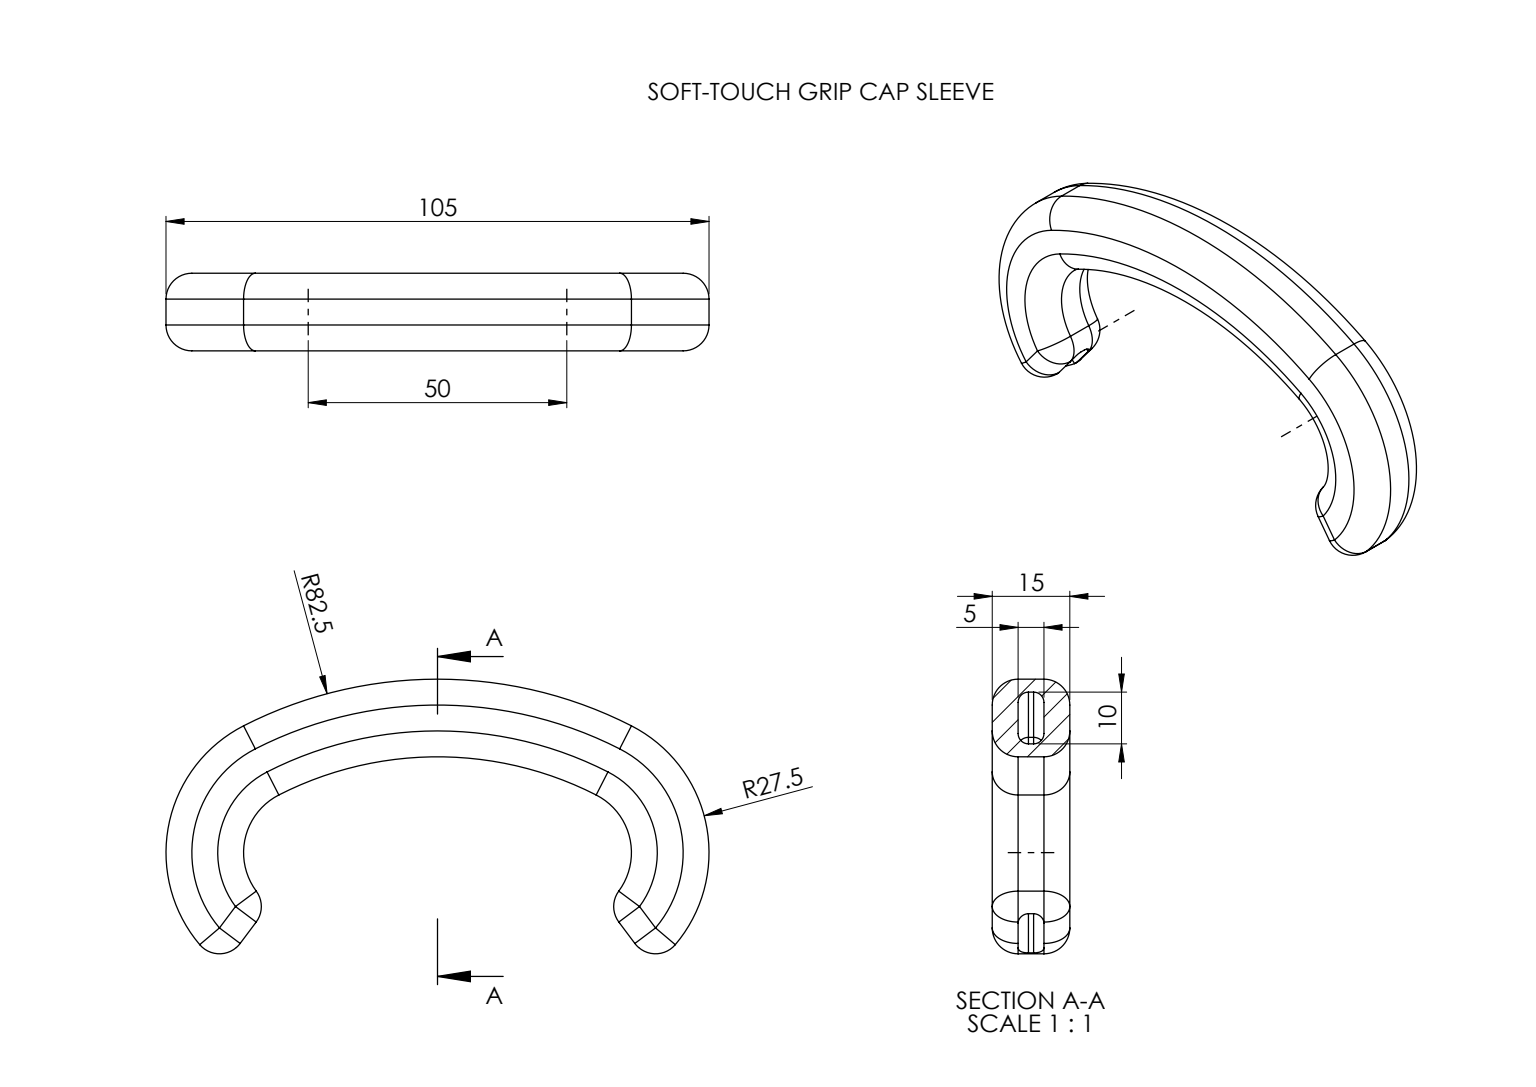
ISO-10303-21;
HEADER;
FILE_DESCRIPTION (('STEP AP214'),
    '1' );
FILE_NAME ('Soft-Touch Grip Cap Sleeve.step',
    '2026-10-08T14:03:35',
    ( '' ),
    ( '' ),
    'SwSTEP 2.0',
    'SolidWorks 2026',
    '' );
FILE_SCHEMA (( 'AUTOMOTIVE_DESIGN' ));
ENDSEC;

DATA;
#11=ORIENTED_EDGE ( 'NONE', *, *, #6966, .F. ) ;
#15=CARTESIAN_POINT ( 'NONE',  ( 35.45454545454547457, 140.4866414850956460, 0.5000000000000000000 ) ) ;
#29=AXIS2_PLACEMENT_3D ( 'NONE', #13329, #9153, #677 ) ;
#40=DIRECTION ( 'NONE',  ( 1.000000000000000000, 8.163404592832038896E-16, 0.000000000000000000 ) ) ;
#44=AXIS2_PLACEMENT_3D ( 'NONE', #13672, #4217, #12871 ) ;
#50=ORIENTED_EDGE ( 'NONE', *, *, #9118, .T. ) ;
#55=B_SPLINE_CURVE_WITH_KNOTS ( 'NONE', 3,
 ( #12024, #7964, #3604, #11191, #2412, #1580, #5937, #3460, #13327, #5788, #331, #6692, #3526, #3678, #4586, #9152 ),
 .UNSPECIFIED., .F., .F.,
 ( 4, 2, 2, 2, 2, 2, 2, 4 ),
 ( 1.967444805616585729E-07, 0.0004077652619395022980, 0.0008153337793984429286, 0.001630470814316324190, 0.002038039331775264550, 0.002445607849234205343, 0.002853176366693145703, 0.003260744884152086496 ),
 .UNSPECIFIED. ) ;
#56=FACE_OUTER_BOUND ( 'NONE', #8177, .T. ) ;
#63=ORIENTED_EDGE ( 'NONE', *, *, #3775, .F. ) ;
#71=ADVANCED_FACE ( 'NONE', ( #7311 ), #13694, .F. ) ;
#72=ORIENTED_EDGE ( 'NONE', *, *, #13139, .F. ) ;
#94=DIRECTION ( 'NONE',  ( 0.000000000000000000, 0.000000000000000000, 1.000000000000000000 ) ) ;
#105=LINE ( 'NONE', #1342, #981 ) ;
#108=CARTESIAN_POINT ( 'NONE',  ( 39.99999999999999289, 120.0000000000000142, -0.5000000000000000000 ) ) ;
#110=ORIENTED_EDGE ( 'NONE', *, *, #13403, .F. ) ;
#115=DIRECTION ( 'NONE',  ( 0.000000000000000000, 0.000000000000000000, 1.000000000000000000 ) ) ;
#121=AXIS2_PLACEMENT_3D ( 'NONE', #813, #875, #8370 ) ;
#138=CARTESIAN_POINT ( 'NONE',  ( -49.99999999999999289, 120.0000000000000142, -0.5000000000000000000 ) ) ;
#139=EDGE_CURVE ( 'NONE', #6890, #1913, #9510, .T. ) ;
#140=FACE_OUTER_BOUND ( 'NONE', #958, .T. ) ;
#148=ORIENTED_EDGE ( 'NONE', *, *, #400, .T. ) ;
#152=DIRECTION ( 'NONE',  ( 1.000000000000000000, 0.000000000000000000, 0.000000000000000000 ) ) ;
#177=ORIENTED_EDGE ( 'NONE', *, *, #6787, .T. ) ;
#187=DIRECTION ( 'NONE',  ( -1.000000000000000000, 0.000000000000000000, 0.000000000000000000 ) ) ;
#196=CARTESIAN_POINT ( 'NONE',  ( 0.000000000000000000, 71.01020514433645303, 7.500000000000000000 ) ) ;
#206=AXIS2_PLACEMENT_3D ( 'NONE', #6163, #5168, #5231 ) ;
#214=VERTEX_POINT ( 'NONE', #5795 ) ;
#224=AXIS2_PLACEMENT_3D ( 'NONE', #10271, #2564, #8106 ) ;
#225=ORIENTED_EDGE ( 'NONE', *, *, #6865, .T. ) ;
#245=AXIS2_PLACEMENT_3D ( 'NONE', #10275, #9294, #13478 ) ;
#272=ORIENTED_EDGE ( 'NONE', *, *, #8857, .F. ) ;
#273=CARTESIAN_POINT ( 'NONE',  ( 35.22727272727274794, 140.0412797136805523, 2.499999999999999556 ) ) ;
#281=EDGE_LOOP ( 'NONE', ( #6165, #11619, #12587 ) ) ;
#289=EDGE_CURVE ( 'NONE', #6878, #1278, #2220, .T. ) ;
#298=AXIS2_PLACEMENT_3D ( 'NONE', #1298, #13105, #6426 ) ;
#303=EDGE_LOOP ( 'NONE', ( #1188, #1446, #12340 ) ) ;
#316=AXIS2_PLACEMENT_3D ( 'NONE', #6986, #3754, #479 ) ;
#330=DIRECTION ( 'NONE',  ( -0.4545454545454531425, -0.8907235428302472391, 0.000000000000000000 ) ) ;
#331=CARTESIAN_POINT ( 'NONE',  ( -39.64259366921353944, 101.1295926276828396, -2.298140577494256931 ) ) ;
#347=AXIS2_PLACEMENT_3D ( 'NONE', #5420, #4428, #2399 ) ;
#351=ORIENTED_EDGE ( 'NONE', *, *, #9753, .F. ) ;
#355=ORIENTED_EDGE ( 'NONE', *, *, #4560, .T. ) ;
#362=AXIS2_PLACEMENT_3D ( 'NONE', #3358, #4277, #12857 ) ;
#365=DIRECTION ( 'NONE',  ( 0.000000000000000000, 0.000000000000000000, 1.000000000000000000 ) ) ;
#369=VERTEX_POINT ( 'NONE', #1786 ) ;
#370=VECTOR ( 'NONE', #9228, 1000.000000000000000 ) ;
#377=DIRECTION ( 'NONE',  ( 0.000000000000000000, 0.000000000000000000, 1.000000000000000000 ) ) ;
#379=EDGE_LOOP ( 'NONE', ( #6863, #5264, #11175, #13440 ) ) ;
#381=AXIS2_PLACEMENT_3D ( 'NONE', #9717, #9650, #7739 ) ;
#382=DIRECTION ( 'NONE',  ( 1.000000000000000000, 0.000000000000000000, 0.000000000000000000 ) ) ;
#397=VERTEX_POINT ( 'NONE', #7385 ) ;
#400=EDGE_CURVE ( 'NONE', #6752, #9552, #11414, .T. ) ;
#406=EDGE_CURVE ( 'NONE', #397, #11234, #4095, .T. ) ;
#410=DIRECTION ( 'NONE',  ( 0.000000000000000000, 0.000000000000000000, 1.000000000000000000 ) ) ;
#414=CARTESIAN_POINT ( 'NONE',  ( 39.06230589874904524, 109.5835921350012683, 2.499999999999999556 ) ) ;
#422=CARTESIAN_POINT ( 'NONE',  ( -39.31777158827905794, 101.3359913474317011, 2.434761661425243418 ) ) ;
#429=DIRECTION ( 'NONE',  ( 0.000000000000000000, 0.000000000000000000, 1.000000000000000000 ) ) ;
#435=VECTOR ( 'NONE', #12367, 1000.000000000000000 ) ;
#436=CARTESIAN_POINT ( 'NONE',  ( -34.25812584745457201, 108.1980041606221192, -0.5000000000000000000 ) ) ;
#448=EDGE_CURVE ( 'NONE', #4575, #2194, #5143, .T. ) ;
#453=DIRECTION ( 'NONE',  ( -0.5999999999999999778, -0.8000000000000000444, 2.220446049250313081E-15 ) ) ;
#467=DIRECTION ( 'NONE',  ( 1.000000000000000000, 0.000000000000000000, 0.000000000000000000 ) ) ;
#478=DIRECTION ( 'NONE',  ( 0.8000000000000000444, 0.5999999999999999778, 0.000000000000000000 ) ) ;
#479=DIRECTION ( 'NONE',  ( 0.7999999999999997113, 0.6000000000000003109, 0.000000000000000000 ) ) ;
#480=EDGE_CURVE ( 'NONE', #8890, #9552, #12010, .T. ) ;
#485=ORIENTED_EDGE ( 'NONE', *, *, #4050, .T. ) ;
#493=EDGE_LOOP ( 'NONE', ( #6586, #7920, #2712, #2336 ) ) ;
#497=AXIS2_PLACEMENT_3D ( 'NONE', #8411, #12702, #2812 ) ;
#499=CARTESIAN_POINT ( 'NONE',  ( -40.33442208022856335, 100.7954446087838107, 1.738653613625529948 ) ) ;
#505=CIRCLE ( 'NONE', #4061, 14.99999999999999112 ) ;
#507=ORIENTED_EDGE ( 'NONE', *, *, #12353, .T. ) ;
#512=CARTESIAN_POINT ( 'NONE',  ( -34.28542361028948449, 108.1059200568371494, -1.103255912984088427 ) ) ;
#516=ORIENTED_EDGE ( 'NONE', *, *, #10493, .T. ) ;
#537=ADVANCED_FACE ( 'NONE', ( #13013 ), #3342, .F. ) ;
#545=ORIENTED_EDGE ( 'NONE', *, *, #289, .F. ) ;
#550=CYLINDRICAL_SURFACE ( 'NONE', #13175, 4.999999999999997335 ) ;
#551=CIRCLE ( 'NONE', #1870, 4.999999999999997335 ) ;
#569=ORIENTED_EDGE ( 'NONE', *, *, #2135, .F. ) ;
#574=CIRCLE ( 'NONE', #8391, 22.49999999999999289 ) ;
#577=SURFACE_STYLE_FILL_AREA ( #12131 ) ;
#578=TOROIDAL_SURFACE ( 'NONE', #8393, 17.49999999999999645, 5.000000000000000000 ) ;
#587=DIRECTION ( 'NONE',  ( -0.000000000000000000, -0.000000000000000000, -1.000000000000000000 ) ) ;
#592=CARTESIAN_POINT ( 'NONE',  ( 34.06230589874905235, 109.5835921350012683, 7.500000000000000000 ) ) ;
#593=CARTESIAN_POINT ( 'NONE',  ( -42.16244658108818300, 105.4500712252157797, -2.499999999999999556 ) ) ;
#596=DIRECTION ( 'NONE',  ( 0.000000000000000000, 1.000000000000000000, 2.775557561562888984E-15 ) ) ;
#599=EDGE_LOOP ( 'NONE', ( #7641, #485, #11774, #148, #4430, #5510 ) ) ;
#602=ORIENTED_EDGE ( 'NONE', *, *, #12372, .T. ) ;
#615=DIRECTION ( 'NONE',  ( -0.000000000000000000, -0.000000000000000000, -1.000000000000000000 ) ) ;
#623=CIRCLE ( 'NONE', #12020, 24.99999999999998934 ) ;
#624=VERTEX_POINT ( 'NONE', #6894 ) ;
#625=CARTESIAN_POINT ( 'NONE',  ( 42.49999999999999289, 120.0000000000000142, -7.500000000000000000 ) ) ;
#629=DIRECTION ( 'NONE',  ( 0.4545454545454531425, -0.8907235428302472391, 0.000000000000000000 ) ) ;
#630=CARTESIAN_POINT ( 'NONE',  ( 0.000000000000000000, 71.01020514433645303, -0.5000000000000000000 ) ) ;
#637=ORIENTED_EDGE ( 'NONE', *, *, #9772, .T. ) ;
#638=ORIENTED_EDGE ( 'NONE', *, *, #13760, .T. ) ;
#639=SURFACE_SIDE_STYLE ('',( #577 ) ) ;
#642=CARTESIAN_POINT ( 'NONE',  ( -39.06230589874905235, 109.5835921350012683, -2.499999999999999556 ) ) ;
#648=DIRECTION ( 'NONE',  ( -4.163336342344333082E-15, 1.000000000000000000, 1.734723475976805615E-16 ) ) ;
#650=CIRCLE ( 'NONE', #9377, 22.49999999999998934 ) ;
#662=CIRCLE ( 'NONE', #206, 4.999999999999996447 ) ;
#668=CARTESIAN_POINT ( 'NONE',  ( 25.00000000000000355, 120.0000000000000142, 2.499999999999999556 ) ) ;
#669=SPHERICAL_SURFACE ( 'NONE', #11083, 5.000000000000000000 ) ;
#676=DIRECTION ( 'NONE',  ( 1.000000000000000000, 3.568574007723717789E-15, 0.000000000000000000 ) ) ;
#677=DIRECTION ( 'NONE',  ( -0.4545454545454531425, -0.8907235428302472391, 0.000000000000000000 ) ) ;
#698=UNCERTAINTY_MEASURE_WITH_UNIT (LENGTH_MEASURE( 1.000000000000000082E-05 ), #1042, 'distance_accuracy_value', 'NONE');
#718=EDGE_CURVE ( 'NONE', #5708, #13751, #11865, .T. ) ;
#727=CARTESIAN_POINT ( 'NONE',  ( 40.81228451836345528, 100.6358150620708329, 0.000000000000000000 ) ) ;
#734=ORIENTED_EDGE ( 'NONE', *, *, #9467, .T. ) ;
#747=CARTESIAN_POINT ( 'NONE',  ( -25.00000000000000355, 120.0000000000000142, -7.500000000000000000 ) ) ;
#749=FACE_OUTER_BOUND ( 'NONE', #779, .T. ) ;
#758=DIRECTION ( 'NONE',  ( -1.000000000000000000, 0.000000000000000000, 0.000000000000000000 ) ) ;
#759=CIRCLE ( 'NONE', #7467, 5.000000000000004441 ) ;
#769=VERTEX_POINT ( 'NONE', #5613 ) ;
#772=CARTESIAN_POINT ( 'NONE',  ( 34.40223077810360763, 107.7696006147693168, 1.740676078835890372 ) ) ;
#779=EDGE_LOOP ( 'NONE', ( #7389, #9473, #2986, #7756 ) ) ;
#780=VERTEX_POINT ( 'NONE', #1145 ) ;
#781=AXIS2_PLACEMENT_3D ( 'NONE', #8266, #3498, #1483 ) ;
#786=ORIENTED_EDGE ( 'NONE', *, *, #3630, .F. ) ;
#787=PLANE ( 'NONE',  #5436 ) ;
#795=CIRCLE ( 'NONE', #347, 22.99999999999999289 ) ;
#797=ORIENTED_EDGE ( 'NONE', *, *, #9932, .F. ) ;
#813=CARTESIAN_POINT ( 'NONE',  ( 42.16244658108818300, 105.4500712252157655, -2.499999999999998668 ) ) ;
#814=DIRECTION ( 'NONE',  ( 0.6000000000000006439, -0.7999999999999996003, -0.000000000000000000 ) ) ;
#817=ORIENTED_EDGE ( 'NONE', *, *, #2795, .F. ) ;
#821=DIRECTION ( 'NONE',  ( 1.000000000000000000, 0.000000000000000000, 0.000000000000000000 ) ) ;
#823=ORIENTED_EDGE ( 'NONE', *, *, #10455, .T. ) ;
#826=CARTESIAN_POINT ( 'NONE',  ( 25.00000000000000355, 120.0000000000000142, -0.5000000000000000000 ) ) ;
#832=DIRECTION ( 'NONE',  ( -0.5999999999999999778, -0.8000000000000000444, -2.220446049250313081E-15 ) ) ;
#840=CARTESIAN_POINT ( 'NONE',  ( 39.06230589874904524, 109.5835921350012683, 7.500000000000000000 ) ) ;
#846=EDGE_LOOP ( 'NONE', ( #3292, #9316, #3361, #5959 ) ) ;
#852=EDGE_LOOP ( 'NONE', ( #11923, #5200, #8675, #11651 ) ) ;
#855=DIRECTION ( 'NONE',  ( 1.086108692045681373E-16, -1.448144922727572616E-16, 1.000000000000000000 ) ) ;
#863=VERTEX_POINT ( 'NONE', #3020 ) ;
#868=DIRECTION ( 'NONE',  ( -1.000000000000000000, 0.000000000000000000, 0.000000000000000000 ) ) ;
#872=ADVANCED_FACE ( 'NONE', ( #11705 ), #7390, .T. ) ;
#874=EDGE_CURVE ( 'NONE', #397, #9139, #6281, .T. ) ;
#875=DIRECTION ( 'NONE',  ( -1.150550675996984260E-16, -1.357138225298697177E-16, 1.000000000000000000 ) ) ;
#892=EDGE_CURVE ( 'NONE', #6479, #12810, #2919, .T. ) ;
#893=CARTESIAN_POINT ( 'NONE',  ( -37.50000000000000000, 120.0000000000000142, -2.499999999999998668 ) ) ;
#895=CARTESIAN_POINT ( 'NONE',  ( 25.00000000000000355, 120.0000000000000142, -2.500000000000000000 ) ) ;
#900=AXIS2_PLACEMENT_3D ( 'NONE', #10736, #8572, #12938 ) ;
#904=ADVANCED_FACE ( 'NONE', ( #11438 ), #13579, .F. ) ;
#905=CIRCLE ( 'NONE', #3346, 5.000000000000000000 ) ;
#909=CARTESIAN_POINT ( 'NONE',  ( 0.000000000000000000, 71.01020514433645303, 7.500000000000000000 ) ) ;
#913=CIRCLE ( 'NONE', #1338, 71.99999999999998579 ) ;
#924=AXIS2_PLACEMENT_3D ( 'NONE', #9907, #12941, #4643 ) ;
#943=DIRECTION ( 'NONE',  ( 1.000000000000000000, 0.000000000000000000, 0.000000000000000000 ) ) ;
#958=EDGE_LOOP ( 'NONE', ( #6961, #7365, #10552, #12347, #1694 ) ) ;
#972=SURFACE_STYLE_USAGE ( .BOTH. , #13448 ) ;
#973=VERTEX_POINT ( 'NONE', #10843 ) ;
#981=VECTOR ( 'NONE', #12875, 999.9999999999998863 ) ;
#995=CARTESIAN_POINT ( 'NONE',  ( -35.06230589874904524, 106.5835921350012825, -2.486789939184904430 ) ) ;
#1003=CARTESIAN_POINT ( 'NONE',  ( 45.97632359910777922, 102.2167537197081657, -2.499999999999998668 ) ) ;
#1011=DIRECTION ( 'NONE',  ( -0.000000000000000000, -0.000000000000000000, -1.000000000000000000 ) ) ;
#1012=CARTESIAN_POINT ( 'NONE',  ( 25.00000000000000355, 120.0000000000000142, 0.5000000000000000000 ) ) ;
#1013=SPHERICAL_SURFACE ( 'NONE', #5602, 5.000000000000000000 ) ;
#1021=TOROIDAL_SURFACE ( 'NONE', #7490, 17.49999999999999289, 5.000000000000000000 ) ;
#1022=ORIENTED_EDGE ( 'NONE', *, *, #13080, .F. ) ;
#1026=DIRECTION ( 'NONE',  ( -1.000000000000000000, 0.000000000000000000, 0.000000000000000000 ) ) ;
#1036=DIRECTION ( 'NONE',  ( 0.000000000000000000, 0.000000000000000000, 1.000000000000000000 ) ) ;
#1042=( LENGTH_UNIT ( ) NAMED_UNIT ( * ) SI_UNIT ( .MILLI., .METRE. ) );
#1050=ADVANCED_FACE ( 'NONE', ( #3213 ), #11773, .T. ) ;
#1058=EDGE_LOOP ( 'NONE', ( #9637, #4616, #13233, #12790 ) ) ;
#1060=DIRECTION ( 'NONE',  ( 1.000000000000000000, 0.000000000000000000, 0.000000000000000000 ) ) ;
#1065=CARTESIAN_POINT ( 'NONE',  ( -34.98870950856983342, 106.6817206552402837, -2.472621650539468696 ) ) ;
#1068=DIRECTION ( 'NONE',  ( -0.5999999999999966471, 0.8000000000000024869, 0.000000000000000000 ) ) ;
#1072=ORIENTED_EDGE ( 'NONE', *, *, #13240, .F. ) ;
#1084=DIRECTION ( 'NONE',  ( 1.000000000000000000, 0.000000000000000000, 0.000000000000000000 ) ) ;
#1085=DIRECTION ( 'NONE',  ( -1.000000000000000000, 0.000000000000000000, 0.000000000000000000 ) ) ;
#1087=CARTESIAN_POINT ( 'NONE',  ( 41.49999999999999289, 98.00000000000001421, 2.499999999999999556 ) ) ;
#1090=ORIENTED_EDGE ( 'NONE', *, *, #5651, .F. ) ;
#1098=CARTESIAN_POINT ( 'NONE',  ( 0.000000000000000000, 71.01020514433645303, 2.499999999999999556 ) ) ;
#1102=CARTESIAN_POINT ( 'NONE',  ( -49.99999999999999289, 120.0000000000000142, 2.500000000000000000 ) ) ;
#1103=EDGE_CURVE ( 'NONE', #769, #13399, #1351, .T. ) ;
#1104=CIRCLE ( 'NONE', #10496, 17.49999999999999289 ) ;
#1109=DIRECTION ( 'NONE',  ( 1.000000000000000000, 0.000000000000000000, 0.000000000000000000 ) ) ;
#1111=CARTESIAN_POINT ( 'NONE',  ( 35.22727272727274084, 140.0412797136805523, 7.500000000000000000 ) ) ;
#1117=ORIENTED_EDGE ( 'NONE', *, *, #5565, .F. ) ;
#1131=CARTESIAN_POINT ( 'NONE',  ( 39.31777158827904373, 101.3359913474316585, -2.434761661425244306 ) ) ;
#1132=DIRECTION ( 'NONE',  ( 1.000000000000000000, 0.000000000000000000, 0.000000000000000000 ) ) ;
#1145=CARTESIAN_POINT ( 'NONE',  ( -42.16244658108818300, 105.4500712252157655, 7.500000000000000000 ) ) ;
#1167=CARTESIAN_POINT ( 'NONE',  ( -25.00000000000000355, 120.0000000000000142, -2.499999999999998668 ) ) ;
#1173=CARTESIAN_POINT ( 'NONE',  ( 40.81228451836346238, 100.6358150620708187, 0.6381026355483961909 ) ) ;
#1188=ORIENTED_EDGE ( 'NONE', *, *, #12808, .T. ) ;
#1193=ADVANCED_FACE ( 'NONE', ( #2400 ), #10537, .F. ) ;
#1196=CARTESIAN_POINT ( 'NONE',  ( -38.89115197531750567, 101.6687180808697519, -2.500000000000000000 ) ) ;
#1200=EDGE_LOOP ( 'NONE', ( #6060, #8837, #10579, #545 ) ) ;
#1203=DIRECTION ( 'NONE',  ( 1.000000000000000000, 0.000000000000000000, 0.000000000000000000 ) ) ;
#1216=CARTESIAN_POINT ( 'NONE',  ( -25.00000000000000355, 120.0000000000000142, -0.5000000000000000000 ) ) ;
#1222=EDGE_LOOP ( 'NONE', ( #13644, #9404, #50, #12785 ) ) ;
#1228=LINE ( 'NONE', #3519, #7961 ) ;
#1236=CARTESIAN_POINT ( 'NONE',  ( 39.06230589874905235, 109.5835921350012683, 7.500000000000000000 ) ) ;
#1238=ADVANCED_FACE ( 'NONE', ( #1643 ), #3580, .T. ) ;
#1239=CARTESIAN_POINT ( 'NONE',  ( -39.06230589874905235, 109.5835921350012683, -7.500000000000000000 ) ) ;
#1241=VECTOR ( 'NONE', #9971, 1000.000000000000000 ) ;
#1268=EDGE_LOOP ( 'NONE', ( #3247, #638, #10126, #9802 ) ) ;
#1278=VERTEX_POINT ( 'NONE', #13536 ) ;
#1283=EDGE_CURVE ( 'NONE', #11234, #8652, #11660, .T. ) ;
#1287=ADVANCED_FACE ( 'NONE', ( #8164 ), #7175, .T. ) ;
#1289=DIRECTION ( 'NONE',  ( -0.000000000000000000, -0.000000000000000000, -1.000000000000000000 ) ) ;
#1294=DIRECTION ( 'NONE',  ( 1.000000000000000000, 0.000000000000000000, 0.000000000000000000 ) ) ;
#1298=CARTESIAN_POINT ( 'NONE',  ( -25.00000000000000355, 120.0000000000000142, 7.500000000000000000 ) ) ;
#1310=ORIENTED_EDGE ( 'NONE', *, *, #12273, .F. ) ;
#1313=CIRCLE ( 'NONE', #12980, 2.000000000000003997 ) ;
#1314=ORIENTED_EDGE ( 'NONE', *, *, #12004, .T. ) ;
#1319=DIRECTION ( 'NONE',  ( 1.000000000000000000, 0.000000000000000000, 0.000000000000000000 ) ) ;
#1325=ORIENTED_EDGE ( 'NONE', *, *, #13518, .F. ) ;
#1338=AXIS2_PLACEMENT_3D ( 'NONE', #7809, #6559, #6766 ) ;
#1342=CARTESIAN_POINT ( 'NONE',  ( 6.999999999999992006, 144.0000000000000284, -2.500000000000000000 ) ) ;
#1347=AXIS2_PLACEMENT_3D ( 'NONE', #10348, #1507, #478 ) ;
#1351=LINE ( 'NONE', #10878, #7831 ) ;
#1352=ORIENTED_EDGE ( 'NONE', *, *, #406, .F. ) ;
#1359=DIRECTION ( 'NONE',  ( 0.000000000000000000, 0.000000000000000000, 1.000000000000000000 ) ) ;
#1361=CIRCLE ( 'NONE', #924, 77.49999999999998579 ) ;
#1364=EDGE_CURVE ( 'NONE', #3469, #6698, #2244, .T. ) ;
#1366=CARTESIAN_POINT ( 'NONE',  ( 40.73187278757659868, 100.6589795836331831, 1.037129925556720789 ) ) ;
#1367=LINE ( 'NONE', #10689, #5432 ) ;
#1370=EDGE_CURVE ( 'NONE', #2025, #13844, #9640, .T. ) ;
#1375=CIRCLE ( 'NONE', #13736, 4.999999999999997335 ) ;
#1385=ORIENTED_EDGE ( 'NONE', *, *, #11158, .T. ) ;
#1396=CARTESIAN_POINT ( 'NONE',  ( -34.31346379765673049, 108.0181378390412732, 1.328939170454191521 ) ) ;
#1400=EDGE_LOOP ( 'NONE', ( #12032, #9944, #11231, #11351, #351 ) ) ;
#1402=CIRCLE ( 'NONE', #3195, 67.49999999999997158 ) ;
#1405=ADVANCED_FACE ( 'NONE', ( #4448 ), #2501, .T. ) ;
#1409=CARTESIAN_POINT ( 'NONE',  ( 0.000000000000000000, 0.000000000000000000, 0.000000000000000000 ) ) ;
#1413=DIRECTION ( 'NONE',  ( -0.000000000000000000, -0.000000000000000000, -1.000000000000000000 ) ) ;
#1422=ORIENTED_EDGE ( 'NONE', *, *, #9090, .F. ) ;
#1430=DIRECTION ( 'NONE',  ( 0.4545454545454531425, 0.8907235428302472391, 0.000000000000000000 ) ) ;
#1435=CARTESIAN_POINT ( 'NONE',  ( 34.50080218526777287, 107.5336849384755737, -2.002074976903565062 ) ) ;
#1436=FACE_OUTER_BOUND ( 'NONE', #12588, .T. ) ;
#1441=DIRECTION ( 'NONE',  ( -0.000000000000000000, -0.000000000000000000, -1.000000000000000000 ) ) ;
#1446=ORIENTED_EDGE ( 'NONE', *, *, #13055, .T. ) ;
#1450=DIRECTION ( 'NONE',  ( -0.000000000000000000, -0.000000000000000000, -1.000000000000000000 ) ) ;
#1451=DIRECTION ( 'NONE',  ( 0.000000000000000000, 0.000000000000000000, 1.000000000000000000 ) ) ;
#1453=CIRCLE ( 'NONE', #2584, 5.000000000000000000 ) ;
#1468=CARTESIAN_POINT ( 'NONE',  ( -34.25812584745450096, 108.1980041606223040, -0.6234894336158697259 ) ) ;
#1471=AXIS2_PLACEMENT_3D ( 'NONE', #642, #2138, #2806 ) ;
#1483=DIRECTION ( 'NONE',  ( -1.000000000000000000, 0.000000000000000000, 0.000000000000000000 ) ) ;
#1492=TOROIDAL_SURFACE ( 'NONE', #5294, 71.99999999999998579, 2.000000000000000000 ) ;
#1498=DIRECTION ( 'NONE',  ( 0.8907235428302464619, -0.4545454545454548079, 4.944508929129155689E-15 ) ) ;
#1499=EDGE_LOOP ( 'NONE', ( #11784, #2877, #786, #13460, #13369 ) ) ;
#1503=EDGE_CURVE ( 'NONE', #3971, #1662, #10328, .T. ) ;
#1507=DIRECTION ( 'NONE',  ( 0.5999999999999999778, -0.8000000000000000444, -2.220446049250313081E-15 ) ) ;
#1508=DIRECTION ( 'NONE',  ( -0.000000000000000000, -0.000000000000000000, -1.000000000000000000 ) ) ;
#1519=EDGE_LOOP ( 'NONE', ( #5605, #7612, #13308, #225, #6231, #6509, #5414, #5521, #11851, #10379 ) ) ;
#1521=CARTESIAN_POINT ( 'NONE',  ( -39.06230589874905235, 109.5835921350012825, 2.499999999999999556 ) ) ;
#1525=CARTESIAN_POINT ( 'NONE',  ( 25.00000000000000355, 120.0000000000000142, 0.5000000000000000000 ) ) ;
#1528=EDGE_LOOP ( 'NONE', ( #12574, #10244, #8782, #6113 ) ) ;
#1530=CARTESIAN_POINT ( 'NONE',  ( -45.97632359910779343, 102.2167537197081799, 7.500000000000000000 ) ) ;
#1532=TOROIDAL_SURFACE ( 'NONE', #8693, 16.99999999999998934, 2.000000000000000000 ) ;
#1536=CARTESIAN_POINT ( 'NONE',  ( -34.37544226909923850, 107.8407100838017385, 1.642507177281961050 ) ) ;
#1540=EDGE_CURVE ( 'NONE', #3748, #6776, #5380, .T. ) ;
#1544=CIRCLE ( 'NONE', #5570, 14.99999999999999112 ) ;
#1554=DIRECTION ( 'NONE',  ( 1.000000000000000000, 0.000000000000000000, 0.000000000000000000 ) ) ;
#1557=VERTEX_POINT ( 'NONE', #4427 ) ;
#1580=CARTESIAN_POINT ( 'NONE',  ( -40.50666510048448288, 100.7305537260640307, -1.531269357928749963 ) ) ;
#1587=VERTEX_POINT ( 'NONE', #11107 ) ;
#1598=AXIS2_PLACEMENT_3D ( 'NONE', #2233, #6519, #152 ) ;
#1602=CARTESIAN_POINT ( 'NONE',  ( 25.00000000000000355, 120.0000000000000142, -2.500000000000000000 ) ) ;
#1610=CYLINDRICAL_SURFACE ( 'NONE', #5111, 4.999999999999997335 ) ;
#1619=DIRECTION ( 'NONE',  ( 1.000000000000000000, 0.000000000000000000, 0.000000000000000000 ) ) ;
#1624=FACE_OUTER_BOUND ( 'NONE', #6612, .T. ) ;
#1641=AXIS2_PLACEMENT_3D ( 'NONE', #4390, #8672, #12972 ) ;
#1643=FACE_OUTER_BOUND ( 'NONE', #12202, .T. ) ;
#1658=CYLINDRICAL_SURFACE ( 'NONE', #316, 5.000000000000001776 ) ;
#1660=ORIENTED_EDGE ( 'NONE', *, *, #6019, .F. ) ;
#1662=VERTEX_POINT ( 'NONE', #6326 ) ;
#1665=CIRCLE ( 'NONE', #11719, 22.49999999999998934 ) ;
#1666=DIRECTION ( 'NONE',  ( 0.000000000000000000, 0.000000000000000000, 1.000000000000000000 ) ) ;
#1669=EDGE_CURVE ( 'NONE', #1961, #973, #9882, .T. ) ;
#1670=DIRECTION ( 'NONE',  ( -0.8907235428302473501, -0.4545454545454531425, -0.000000000000000000 ) ) ;
#1673=UNCERTAINTY_MEASURE_WITH_UNIT (LENGTH_MEASURE( 1.000000000000000082E-05 ), #11236, 'distance_accuracy_value', 'NONE');
#1685=CARTESIAN_POINT ( 'NONE',  ( -35.06230589874904524, 106.5835921350012825, 2.486789939184904430 ) ) ;
#1688=EDGE_LOOP ( 'NONE', ( #13191, #9298, #10352, #13341 ) ) ;
#1690=( GEOMETRIC_REPRESENTATION_CONTEXT ( 3 ) GLOBAL_UNCERTAINTY_ASSIGNED_CONTEXT ( ( #1673 ) ) GLOBAL_UNIT_ASSIGNED_CONTEXT ( ( #11236, #12500, #12288 ) ) REPRESENTATION_CONTEXT ( 'NONE', 'WORKASPACE' ) );
#1694=ORIENTED_EDGE ( 'NONE', *, *, #12378, .F. ) ;
#1702=STYLED_ITEM ( 'NONE', ( #12834 ), #5722 ) ;
#1704=CIRCLE ( 'NONE', #13621, 24.99999999999998934 ) ;
#1707=EDGE_LOOP ( 'NONE', ( #11988, #1976, #8800, #9233 ) ) ;
#1715=DIRECTION ( 'NONE',  ( 0.000000000000000000, -1.000000000000000000, 0.000000000000000000 ) ) ;
#1726=ORIENTED_EDGE ( 'NONE', *, *, #10712, .T. ) ;
#1730=EDGE_CURVE ( 'NONE', #13845, #5632, #4275, .T. ) ;
#1731=EDGE_LOOP ( 'NONE', ( #2801, #8861, #13593, #2533 ) ) ;
#1732=ORIENTED_EDGE ( 'NONE', *, *, #10569, .F. ) ;
#1735=CARTESIAN_POINT ( 'NONE',  ( -32.95454545454546746, 135.5876619995293311, -7.500000000000000000 ) ) ;
#1744=B_SPLINE_CURVE_WITH_KNOTS ( 'NONE', 3,
 ( #11710, #3219, #13065, #1131, #13856, #6523, #2102, #11642, #5388, #11844, #10655, #2041, #10848, #2237, #9675, #8686 ),
 .UNSPECIFIED., .F., .F.,
 ( 4, 2, 2, 2, 2, 2, 2, 4 ),
 ( 0.001123485749927446119, 0.001530777205506870077, 0.001938068661086294036, 0.002345360116665717778, 0.002752651572245141953, 0.003159943027824565695, 0.003567234483403990304, 0.004381817394562847329 ),
 .UNSPECIFIED. ) ;
#1747=DIRECTION ( 'NONE',  ( 0.000000000000000000, 0.000000000000000000, 1.000000000000000000 ) ) ;
#1750=EDGE_CURVE ( 'NONE', #6075, #13845, #11971, .T. ) ;
#1754=ADVANCED_FACE ( 'NONE', ( #12267 ), #3629, .F. ) ;
#1758=ORIENTED_EDGE ( 'NONE', *, *, #8328, .T. ) ;
#1781=AXIS2_PLACEMENT_3D ( 'NONE', #10677, #8646, #2395 ) ;
#1786=CARTESIAN_POINT ( 'NONE',  ( -35.20000000000000995, 106.3999999999999915, -2.500000000000000000 ) ) ;
#1794=EDGE_CURVE ( 'NONE', #4611, #2641, #8895, .T. ) ;
#1809=EDGE_CURVE ( 'NONE', #6479, #12375, #6718, .T. ) ;
#1812=ORIENTED_EDGE ( 'NONE', *, *, #5748, .T. ) ;
#1831=ORIENTED_EDGE ( 'NONE', *, *, #6798, .T. ) ;
#1833=VERTEX_POINT ( 'NONE', #13563 ) ;
#1836=DIRECTION ( 'NONE',  ( 0.7999999999999996003, -0.6000000000000007550, 0.000000000000000000 ) ) ;
#1843=ORIENTED_EDGE ( 'NONE', *, *, #5247, .T. ) ;
#1844=CIRCLE ( 'NONE', #9670, 2.000000000000003997 ) ;
#1852=DIRECTION ( 'NONE',  ( 1.000000000000000000, 0.000000000000000000, 0.000000000000000000 ) ) ;
#1853=CARTESIAN_POINT ( 'NONE',  ( 39.06230589874905235, 109.5835921350012683, 2.499999999999999556 ) ) ;
#1858=AXIS2_PLACEMENT_3D ( 'NONE', #13495, #6022, #2582 ) ;
#1861=CARTESIAN_POINT ( 'NONE',  ( 25.00000000000000355, 120.0000000000000142, 0.5000000000000000000 ) ) ;
#1866=DIRECTION ( 'NONE',  ( -0.000000000000000000, -0.000000000000000000, -1.000000000000000000 ) ) ;
#1870=AXIS2_PLACEMENT_3D ( 'NONE', #3571, #12221, #11235 ) ;
#1877=AXIS2_PLACEMENT_3D ( 'NONE', #2612, #4708, #3983 ) ;
#1884=TOROIDAL_SURFACE ( 'NONE', #8383, 77.49999999999998579, 5.000000000000000000 ) ;
#1888=ORIENTED_EDGE ( 'NONE', *, *, #448, .T. ) ;
#1896=CIRCLE ( 'NONE', #5250, 14.99999999999998934 ) ;
#1898=ORIENTED_EDGE ( 'NONE', *, *, #3506, .T. ) ;
#1908=CARTESIAN_POINT ( 'NONE',  ( 35.20000000000002416, 106.3999999999999915, 0.5000000000000000000 ) ) ;
#1913=VERTEX_POINT ( 'NONE', #12437 ) ;
#1917=DIRECTION ( 'NONE',  ( -0.000000000000000000, -0.000000000000000000, -1.000000000000000000 ) ) ;
#1920=CARTESIAN_POINT ( 'NONE',  ( 39.06230589874904524, 109.5835921350012683, 2.499999999999999556 ) ) ;
#1928=DIRECTION ( 'NONE',  ( -0.4545454545454558626, 0.8907235428302457958, 0.000000000000000000 ) ) ;
#1937=CARTESIAN_POINT ( 'NONE',  ( -35.06230589874904524, 106.5835921350012825, 2.486789939184904430 ) ) ;
#1961=VERTEX_POINT ( 'NONE', #13311 ) ;
#1976=ORIENTED_EDGE ( 'NONE', *, *, #2575, .T. ) ;
#1986=FACE_OUTER_BOUND ( 'NONE', #12322, .T. ) ;
#1997=DIRECTION ( 'NONE',  ( 0.000000000000000000, 0.000000000000000000, 1.000000000000000000 ) ) ;
#2002=ORIENTED_EDGE ( 'NONE', *, *, #12623, .T. ) ;
#2014=AXIS2_PLACEMENT_3D ( 'NONE', #9048, #7925, #2598 ) ;
#2017=CARTESIAN_POINT ( 'NONE',  ( 39.99999999999999289, 120.0000000000000142, 0.5000000000000000000 ) ) ;
#2018=CIRCLE ( 'NONE', #9858, 2.000000000000000000 ) ;
#2019=AXIS2_PLACEMENT_3D ( 'NONE', #8212, #2034, #9263 ) ;
#2025=VERTEX_POINT ( 'NONE', #7606 ) ;
#2034=DIRECTION ( 'NONE',  ( -0.5952233065713573579, -0.8035603370713738647, -3.056366244416775696E-15 ) ) ;
#2035=ORIENTED_EDGE ( 'NONE', *, *, #400, .F. ) ;
#2037=TOROIDAL_SURFACE ( 'NONE', #5612, 22.99999999999999289, 2.000000000000000000 ) ;
#2041=CARTESIAN_POINT ( 'NONE',  ( 40.49366238756158509, 100.7360090884195216, -1.526167340029800146 ) ) ;
#2055=DIRECTION ( 'NONE',  ( 1.000000000000000000, 0.000000000000000000, 0.000000000000000000 ) ) ;
#2057=CARTESIAN_POINT ( 'NONE',  ( 35.06230589874905945, 106.5835921350012683, 7.500000000000000000 ) ) ;
#2059=DIRECTION ( 'NONE',  ( -0.000000000000000000, -0.000000000000000000, -1.000000000000000000 ) ) ;
#2060=CIRCLE ( 'NONE', #9898, 2.000000000000007105 ) ;
#2061=CARTESIAN_POINT ( 'NONE',  ( 35.06230589874905945, 106.5835921350012683, 7.500000000000000000 ) ) ;
#2064=DIRECTION ( 'NONE',  ( -1.150550675996984260E-16, -1.357138225298697177E-16, 1.000000000000000000 ) ) ;
#2065=EDGE_CURVE ( 'NONE', #10096, #2984, #905, .T. ) ;
#2066=EDGE_LOOP ( 'NONE', ( #6390, #569, #4598, #7412, #5148 ) ) ;
#2067=FACE_OUTER_BOUND ( 'NONE', #13413, .T. ) ;
#2070=CARTESIAN_POINT ( 'NONE',  ( -25.00000000000000355, 120.0000000000000142, 2.500000000000000000 ) ) ;
#2071=EDGE_CURVE ( 'NONE', #4214, #5708, #9630, .T. ) ;
#2076=DIRECTION ( 'NONE',  ( 0.8000000000000000444, -0.5999999999999999778, 0.000000000000000000 ) ) ;
#2091=ORIENTED_EDGE ( 'NONE', *, *, #2398, .T. ) ;
#2096=DIRECTION ( 'NONE',  ( 0.000000000000000000, 0.000000000000000000, 1.000000000000000000 ) ) ;
#2097=VERTEX_POINT ( 'NONE', #4224 ) ;
#2102=CARTESIAN_POINT ( 'NONE',  ( 39.75092559767094258, 101.0685047868945929, -2.236846530894074814 ) ) ;
#2109=CIRCLE ( 'NONE', #4822, 27.49999999999998579 ) ;
#2112=CARTESIAN_POINT ( 'NONE',  ( -42.16244658108818300, 105.4500712252157655, -7.500000000000000000 ) ) ;
#2115=DIRECTION ( 'NONE',  ( 1.000000000000000000, 0.000000000000000000, 0.000000000000000000 ) ) ;
#2116=CIRCLE ( 'NONE', #12673, 5.000000000000001776 ) ;
#2117=CARTESIAN_POINT ( 'NONE',  ( 42.49999999999999289, 120.0000000000000142, -2.499999999999998668 ) ) ;
#2119=EDGE_CURVE ( 'NONE', #11283, #369, #12560, .T. ) ;
#2121=AXIS2_PLACEMENT_3D ( 'NONE', #3251, #7526, #3314 ) ;
#2122=FACE_OUTER_BOUND ( 'NONE', #10513, .T. ) ;
#2129=ORIENTED_EDGE ( 'NONE', *, *, #1103, .T. ) ;
#2135=EDGE_CURVE ( 'NONE', #1587, #8382, #3177, .T. ) ;
#2138=DIRECTION ( 'NONE',  ( 0.000000000000000000, 1.000000000000000000, 0.000000000000000000 ) ) ;
#2143=CIRCLE ( 'NONE', #121, 5.000000000000004441 ) ;
#2161=ORIENTED_EDGE ( 'NONE', *, *, #10712, .F. ) ;
#2162=CARTESIAN_POINT ( 'NONE',  ( -42.16244658108818300, 105.4500712252157655, -2.499999999999999556 ) ) ;
#2165=CARTESIAN_POINT ( 'NONE',  ( -32.50000000000000000, 110.0000000000000142, 7.500000000000000000 ) ) ;
#2172=ORIENTED_EDGE ( 'NONE', *, *, #3775, .T. ) ;
#2176=DIRECTION ( 'NONE',  ( 1.000000000000000000, 0.000000000000000000, 0.000000000000000000 ) ) ;
#2188=DIRECTION ( 'NONE',  ( 1.000000000000000000, 0.000000000000000000, 0.000000000000000000 ) ) ;
#2194=VERTEX_POINT ( 'NONE', #108 ) ;
#2203=CARTESIAN_POINT ( 'NONE',  ( -32.95454545454546746, 135.5876619995293311, 2.499999999999999556 ) ) ;
#2205=CARTESIAN_POINT ( 'NONE',  ( 39.95570474821488460, 100.9618745346225523, 2.097587229781389340 ) ) ;
#2208=TOROIDAL_SURFACE ( 'NONE', #10924, 22.99999999999999289, 2.000000000000000000 ) ;
#2210=CLOSED_SHELL ( 'NONE', ( #1193, #13062, #3042, #5170, #9600, #904, #13357, #10841, #5079, #1287, #8147, #1754, #13816, #12553, #3074, #3880, #4363, #6608, #5498, #12189, #6358, #13551, #1405, #5948, #7195, #10378, #4308, #11825, #7549, #872, #4835, #2576, #4664, #9877, #13684, #8115, #9780, #1050, #6606, #12109, #10292, #11732, #4206, #5152, #8485, #9353, #8225, #4452, #5003, #13186, #6597, #3776, #1238, #2494, #6120, #8591, #9805, #13267, #10474, #12422, #5660, #537, #12969, #8967, #8421, #11407, #7917, #71, #6262, #3412, #13662, #4752, #9281 ) ) ;
#2212=SHAPE_REPRESENTATION_RELATIONSHIP ( 'NONE' , 'NONE' ,  #5134, #5722 ) ;
#2215=CARTESIAN_POINT ( 'NONE',  ( 38.89115197531749857, 101.6687180808697377, -2.500000000000000000 ) ) ;
#2220=CIRCLE ( 'NONE', #11852, 24.99999999999998934 ) ;
#2228=AXIS2_PLACEMENT_3D ( 'NONE', #3934, #11506, #12497 ) ;
#2233=CARTESIAN_POINT ( 'NONE',  ( -25.00000000000000355, 120.0000000000000142, 2.499999999999999556 ) ) ;
#2237=CARTESIAN_POINT ( 'NONE',  ( 40.74280923682186284, 100.6542365527006098, -1.046903941091064327 ) ) ;
#2244=CIRCLE ( 'NONE', #5606, 17.49999999999999289 ) ;
#2249=AXIS2_PLACEMENT_3D ( 'NONE', #4293, #6143, #1084 ) ;
#2271=DIRECTION ( 'NONE',  ( 0.8907235428302473501, -0.4545454545454531425, 0.000000000000000000 ) ) ;
#2272=EDGE_LOOP ( 'NONE', ( #10595, #6257, #8125, #2688 ) ) ;
#2279=FACE_OUTER_BOUND ( 'NONE', #12166, .T. ) ;
#2280=CARTESIAN_POINT ( 'NONE',  ( 39.74871155318042781, 101.0697170996391492, 2.238193420436154657 ) ) ;
#2294=ORIENTED_EDGE ( 'NONE', *, *, #1730, .F. ) ;
#2300=CARTESIAN_POINT ( 'NONE',  ( -34.31344059123750156, 108.0182175921208909, -1.328634118392872043 ) ) ;
#2308=ORIENTED_EDGE ( 'NONE', *, *, #5750, .T. ) ;
#2310=EDGE_CURVE ( 'NONE', #863, #11542, #10737, .T. ) ;
#2312=CARTESIAN_POINT ( 'NONE',  ( 34.06230589874905235, 109.5835921350012683, -2.499999999999999112 ) ) ;
#2313=DIRECTION ( 'NONE',  ( -0.000000000000000000, -0.000000000000000000, -1.000000000000000000 ) ) ;
#2318=LINE ( 'NONE', #9686, #1241 ) ;
#2319=DIRECTION ( 'NONE',  ( 0.000000000000000000, 0.000000000000000000, 1.000000000000000000 ) ) ;
#2333=ORIENTED_EDGE ( 'NONE', *, *, #8076, .F. ) ;
#2335=CARTESIAN_POINT ( 'NONE',  ( 25.00000000000000355, 120.0000000000000142, 7.500000000000000000 ) ) ;
#2336=ORIENTED_EDGE ( 'NONE', *, *, #7773, .F. ) ;
#2337=DIRECTION ( 'NONE',  ( -1.000000000000000000, 0.000000000000000000, 0.000000000000000000 ) ) ;
#2338=AXIS2_PLACEMENT_3D ( 'NONE', #13400, #8030, #12309 ) ;
#2345=LINE ( 'NONE', #6357, #5557 ) ;
#2350=DIRECTION ( 'NONE',  ( -0.000000000000000000, -0.000000000000000000, -1.000000000000000000 ) ) ;
#2356=COLOUR_RGB ( '', 0.66274510, 0.83137255, 0.94901961) ;
#2363=EDGE_CURVE ( 'NONE', #10350, #13844, #8301, .T. ) ;
#2367=DIRECTION ( 'NONE',  ( 1.000000000000000000, 0.000000000000000000, 0.000000000000000000 ) ) ;
#2368=DIRECTION ( 'NONE',  ( -0.000000000000000000, -0.000000000000000000, -1.000000000000000000 ) ) ;
#2381=EDGE_LOOP ( 'NONE', ( #6923, #11451, #4968, #6883, #1090 ) ) ;
#2384=CARTESIAN_POINT ( 'NONE',  ( -25.00000000000000355, 120.0000000000000142, 0.5000000000000000000 ) ) ;
#2395=DIRECTION ( 'NONE',  ( 1.000000000000000000, 0.000000000000000000, 0.000000000000000000 ) ) ;
#2398=EDGE_CURVE ( 'NONE', #11283, #10135, #10965, .T. ) ;
#2399=DIRECTION ( 'NONE',  ( 1.000000000000000000, 0.000000000000000000, 0.000000000000000000 ) ) ;
#2400=FACE_OUTER_BOUND ( 'NONE', #11892, .T. ) ;
#2402=ORIENTED_EDGE ( 'NONE', *, *, #3002, .T. ) ;
#2409=CARTESIAN_POINT ( 'NONE',  ( 34.27497211191903403, 108.1406786207261916, -0.9834270823685519192 ) ) ;
#2412=CARTESIAN_POINT ( 'NONE',  ( -40.68412312724079527, 100.6732077982501181, -1.167148848990504639 ) ) ;
#2425=DIRECTION ( 'NONE',  ( 0.8907235428302465730, -0.4545454545454549189, 2.472254464564578633E-15 ) ) ;
#2429=VECTOR ( 'NONE', #11889, 1000.000000000000000 ) ;
#2433=EDGE_LOOP ( 'NONE', ( #6823, #10972, #2035, #11618 ) ) ;
#2435=AXIS2_PLACEMENT_3D ( 'NONE', #6592, #4344, #5337 ) ;
#2436=VERTEX_POINT ( 'NONE', #11479 ) ;
#2440=CARTESIAN_POINT ( 'NONE',  ( 0.000000000000000000, 71.01020514433645303, -0.5000000000000000000 ) ) ;
#2447=FACE_OUTER_BOUND ( 'NONE', #852, .T. ) ;
#2453=AXIS2_PLACEMENT_3D ( 'NONE', #4488, #2313, #5470 ) ;
#2455=SPHERICAL_SURFACE ( 'NONE', #10720, 5.000000000000000000 ) ;
#2460=DIRECTION ( 'NONE',  ( 1.000000000000000000, 0.000000000000000000, 0.000000000000000000 ) ) ;
#2464=CARTESIAN_POINT ( 'NONE',  ( 37.50000000000002132, 144.4948974278317735, 7.500000000000000000 ) ) ;
#2467=VECTOR ( 'NONE', #13179, 999.9999999999998863 ) ;
#2468=CARTESIAN_POINT ( 'NONE',  ( 0.000000000000000000, 71.01020514433645303, -0.5000000000000000000 ) ) ;
#2476=STYLED_ITEM ( 'NONE', ( #6796 ), #3316 ) ;
#2477=AXIS2_PLACEMENT_3D ( 'NONE', #196, #6633, #8880 ) ;
#2487=CARTESIAN_POINT ( 'NONE',  ( 34.26147919318644597, 108.1862277804541606, -0.7448039452652778225 ) ) ;
#2488=DIRECTION ( 'NONE',  ( -0.000000000000000000, -0.000000000000000000, -1.000000000000000000 ) ) ;
#2494=ADVANCED_FACE ( 'NONE', ( #8592 ), #11547, .F. ) ;
#2496=SPHERICAL_SURFACE ( 'NONE', #6245, 5.000000000000000000 ) ;
#2499=CARTESIAN_POINT ( 'NONE',  ( 25.00000000000000355, 120.0000000000000142, 0.5000000000000000000 ) ) ;
#2501=CYLINDRICAL_SURFACE ( 'NONE', #2477, 82.49999999999998579 ) ;
#2508=CARTESIAN_POINT ( 'NONE',  ( -40.81228451836347659, 100.6358150620708471, 0.5000000000000000000 ) ) ;
#2513=VECTOR ( 'NONE', #6343, 1000.000000000000000 ) ;
#2515=VERTEX_POINT ( 'NONE', #893 ) ;
#2519=SURFACE_STYLE_USAGE ( .BOTH. , #639 ) ;
#2522=FACE_OUTER_BOUND ( 'NONE', #493, .T. ) ;
#2523=CARTESIAN_POINT ( 'NONE',  ( 34.25812584745457201, 108.1980041606221050, -0.5000000000000000000 ) ) ;
#2533=ORIENTED_EDGE ( 'NONE', *, *, #9256, .F. ) ;
#2538=CIRCLE ( 'NONE', #4317, 4.999999999999997335 ) ;
#2540=DIRECTION ( 'NONE',  ( 1.067526471530071686E-16, 1.423368628706762330E-16, 1.000000000000000000 ) ) ;
#2543=FACE_OUTER_BOUND ( 'NONE', #2433, .T. ) ;
#2560=CARTESIAN_POINT ( 'NONE',  ( 0.000000000000000000, 71.01020514433645303, 2.500000000000000000 ) ) ;
#2564=DIRECTION ( 'NONE',  ( 0.000000000000000000, 0.000000000000000000, 1.000000000000000000 ) ) ;
#2568=DIRECTION ( 'NONE',  ( -0.000000000000000000, 1.000000000000000000, 0.000000000000000000 ) ) ;
#2573=VERTEX_POINT ( 'NONE', #10686 ) ;
#2574=CARTESIAN_POINT ( 'NONE',  ( 47.49999999999999289, 120.0000000000000142, -7.500000000000000000 ) ) ;
#2575=EDGE_CURVE ( 'NONE', #769, #3876, #4714, .T. ) ;
#2576=ADVANCED_FACE ( 'NONE', ( #56 ), #9850, .T. ) ;
#2581=EDGE_CURVE ( 'NONE', #1833, #12810, #9999, .T. ) ;
#2582=DIRECTION ( 'NONE',  ( 0.000000000000000000, 0.000000000000000000, -1.000000000000000000 ) ) ;
#2584=AXIS2_PLACEMENT_3D ( 'NONE', #13470, #1715, #12446 ) ;
#2590=EDGE_CURVE ( 'NONE', #2515, #2097, #6291, .T. ) ;
#2591=AXIS2_PLACEMENT_3D ( 'NONE', #12724, #1917, #9425 ) ;
#2592=EDGE_CURVE ( 'NONE', #7525, #11283, #913, .T. ) ;
#2598=DIRECTION ( 'NONE',  ( 0.7627754036039178231, -0.6466635011015234857, 0.000000000000000000 ) ) ;
#2600=CARTESIAN_POINT ( 'NONE',  ( -34.28525802518650067, 108.1064455385057670, 1.101804919165826790 ) ) ;
#2612=CARTESIAN_POINT ( 'NONE',  ( 42.16244658108817589, 105.4500712252157655, 2.499999999999999556 ) ) ;
#2629=ORIENTED_EDGE ( 'NONE', *, *, #7360, .F. ) ;
#2641=VERTEX_POINT ( 'NONE', #7532 ) ;
#2653=EDGE_CURVE ( 'NONE', #863, #9139, #8087, .T. ) ;
#2657=DIRECTION ( 'NONE',  ( -0.000000000000000000, -0.000000000000000000, -1.000000000000000000 ) ) ;
#2663=CARTESIAN_POINT ( 'NONE',  ( -34.26155123102907396, 108.1859746833188041, -0.7471162051235282764 ) ) ;
#2679=FILL_AREA_STYLE ('',( #9200 ) ) ;
#2685=AXIS2_PLACEMENT_3D ( 'NONE', #13873, #11664, #9292 ) ;
#2687=DIRECTION ( 'NONE',  ( 0.7999999999999999334, -0.6000000000000001998, 0.000000000000000000 ) ) ;
#2688=ORIENTED_EDGE ( 'NONE', *, *, #892, .F. ) ;
#2701=CARTESIAN_POINT ( 'NONE',  ( 25.00000000000000355, 120.0000000000000142, 7.500000000000000000 ) ) ;
#2707=DIRECTION ( 'NONE',  ( -0.4545454545454548634, 0.8907235428302464619, 0.000000000000000000 ) ) ;
#2712=ORIENTED_EDGE ( 'NONE', *, *, #7531, .T. ) ;
#2722=VECTOR ( 'NONE', #12127, 999.9999999999998863 ) ;
#2737=EDGE_CURVE ( 'NONE', #2641, #3010, #8073, .T. ) ;
#2745=CARTESIAN_POINT ( 'NONE',  ( -25.00000000000000355, 120.0000000000000142, 0.5000000000000000000 ) ) ;
#2747=ORIENTED_EDGE ( 'NONE', *, *, #6781, .F. ) ;
#2749=EDGE_CURVE ( 'NONE', #11361, #6776, #2018, .T. ) ;
#2752=DIRECTION ( 'NONE',  ( 0.000000000000000000, 0.000000000000000000, 1.000000000000000000 ) ) ;
#2762=VERTEX_POINT ( 'NONE', #10735 ) ;
#2770=CIRCLE ( 'NONE', #10797, 16.99999999999998934 ) ;
#2785=DIRECTION ( 'NONE',  ( 1.000000000000000000, 0.000000000000000000, 0.000000000000000000 ) ) ;
#2793=DIRECTION ( 'NONE',  ( 1.000000000000000000, 3.636937494461720708E-15, 0.000000000000000000 ) ) ;
#2794=CARTESIAN_POINT ( 'NONE',  ( -40.81228451836656745, 100.6358150620699519, 0.7758357214534903346 ) ) ;
#2795=EDGE_CURVE ( 'NONE', #5632, #5338, #5591, .T. ) ;
#2798=VECTOR ( 'NONE', #3187, 1000.000000000000000 ) ;
#2801=ORIENTED_EDGE ( 'NONE', *, *, #7321, .F. ) ;
#2806=DIRECTION ( 'NONE',  ( -1.000000000000000000, 0.000000000000000000, 0.000000000000000000 ) ) ;
#2812=DIRECTION ( 'NONE',  ( 0.8000000000000012657, -0.5999999999999982014, 0.000000000000000000 ) ) ;
#2813=CIRCLE ( 'NONE', #10639, 1.999999999999998890 ) ;
#2829=VERTEX_POINT ( 'NONE', #12225 ) ;
#2830=EDGE_CURVE ( 'NONE', #4611, #5338, #7408, .T. ) ;
#2836=FACE_OUTER_BOUND ( 'NONE', #4704, .T. ) ;
#2852=EDGE_CURVE ( 'NONE', #6776, #9459, #5190, .T. ) ;
#2857=DIRECTION ( 'NONE',  ( 1.000000000000000000, 5.551115123125788224E-15, 0.000000000000000000 ) ) ;
#2859=CARTESIAN_POINT ( 'NONE',  ( -30.68181818181819054, 131.1340442853780814, 2.499999999999999556 ) ) ;
#2875=AXIS2_PLACEMENT_3D ( 'NONE', #7353, #6191, #1836 ) ;
#2877=ORIENTED_EDGE ( 'NONE', *, *, #6865, .F. ) ;
#2887=B_SPLINE_CURVE_WITH_KNOTS ( 'NONE', 3,
 ( #13286, #12209, #10995, #3635, #2600, #1396, #6876, #1536, #5678, #4623, #3558, #13641, #4906, #10238, #12487, #1685 ),
 .UNSPECIFIED., .F., .F.,
 ( 4, 2, 2, 2, 2, 2, 2, 4 ),
 ( 1.969947839882000721E-07, 0.0003650593540107636178, 0.0007299217132375390368, 0.001094784072464314618, 0.001459646431691089983, 0.001824508790917865131, 0.002189371150144640930, 0.002919095868598201200 ),
 .UNSPECIFIED. ) ;
#2900=DIRECTION ( 'NONE',  ( 1.000000000000000000, 0.000000000000000000, 0.000000000000000000 ) ) ;
#2907=DIRECTION ( 'NONE',  ( 0.000000000000000000, 0.000000000000000000, 1.000000000000000000 ) ) ;
#2912=CARTESIAN_POINT ( 'NONE',  ( 52.49999999999999289, 120.0000000000000142, -2.499999999999998668 ) ) ;
#2913=ORIENTED_EDGE ( 'NONE', *, *, #8360, .F. ) ;
#2919=CIRCLE ( 'NONE', #2019, 5.000000000000000888 ) ;
#2920=EDGE_LOOP ( 'NONE', ( #10332, #13431, #1314, #12772 ) ) ;
#2921=DIRECTION ( 'NONE',  ( 0.6000000000000024203, -0.7999999999999982681, -0.000000000000000000 ) ) ;
#2925=TOROIDAL_SURFACE ( 'NONE', #6717, 17.49999999999999289, 5.000000000000000000 ) ;
#2945=CARTESIAN_POINT ( 'NONE',  ( 34.31344059123750867, 108.0182175921209051, 1.328634118392873598 ) ) ;
#2954=ORIENTED_EDGE ( 'NONE', *, *, #12971, .F. ) ;
#2956=VERTEX_POINT ( 'NONE', #7318 ) ;
#2961=FACE_OUTER_BOUND ( 'NONE', #10260, .T. ) ;
#2975=DIRECTION ( 'NONE',  ( 0.000000000000000000, 0.000000000000000000, 1.000000000000000000 ) ) ;
#2984=VERTEX_POINT ( 'NONE', #2912 ) ;
#2986=ORIENTED_EDGE ( 'NONE', *, *, #7531, .F. ) ;
#2988=CARTESIAN_POINT ( 'NONE',  ( 25.00000000000000355, 120.0000000000000142, -0.5000000000000000000 ) ) ;
#3000=CIRCLE ( 'NONE', #9053, 4.999999999999998224 ) ;
#3002=EDGE_CURVE ( 'NONE', #6314, #8647, #2060, .T. ) ;
#3005=CARTESIAN_POINT ( 'NONE',  ( 34.98870950856983342, 106.6817206552402268, 2.472621650539469584 ) ) ;
#3008=CARTESIAN_POINT ( 'NONE',  ( 48.00000000000000000, 120.0000000000000142, -0.5000000000000000000 ) ) ;
#3010=VERTEX_POINT ( 'NONE', #9437 ) ;
#3014=VECTOR ( 'NONE', #12905, 1000.000000000000000 ) ;
#3020=CARTESIAN_POINT ( 'NONE',  ( -32.95454545454546746, 135.5876619995293311, 7.500000000000000000 ) ) ;
#3023=EDGE_CURVE ( 'NONE', #8382, #5087, #4161, .T. ) ;
#3034=EDGE_LOOP ( 'NONE', ( #11101, #4938, #7770, #12252, #1758, #516 ) ) ;
#3038=LINE ( 'NONE', #4080, #12312 ) ;
#3042=ADVANCED_FACE ( 'NONE', ( #7835 ), #7877, .F. ) ;
#3044=LINE ( 'NONE', #10672, #8500 ) ;
#3070=TOROIDAL_SURFACE ( 'NONE', #6646, 22.99999999999999289, 2.000000000000000000 ) ;
#3074=ADVANCED_FACE ( 'NONE', ( #4989 ), #8231, .T. ) ;
#3077=ORIENTED_EDGE ( 'NONE', *, *, #3701, .T. ) ;
#3081=DIRECTION ( 'NONE',  ( 1.000000000000000000, 0.000000000000000000, 0.000000000000000000 ) ) ;
#3096=EDGE_CURVE ( 'NONE', #9459, #12157, #1844, .T. ) ;
#3099=DIRECTION ( 'NONE',  ( 0.8907235428302464619, 0.4545454545454548079, 0.000000000000000000 ) ) ;
#3102=CARTESIAN_POINT ( 'NONE',  ( 0.000000000000000000, 71.01020514433645303, 2.499999999999999556 ) ) ;
#3115=ORIENTED_EDGE ( 'NONE', *, *, #12623, .F. ) ;
#3117=FACE_OUTER_BOUND ( 'NONE', #10053, .T. ) ;
#3138=ORIENTED_EDGE ( 'NONE', *, *, #3565, .F. ) ;
#3150=AXIS2_PLACEMENT_3D ( 'NONE', #12021, #5307, #9659 ) ;
#3159=AXIS2_PLACEMENT_3D ( 'NONE', #593, #2540, #4711 ) ;
#3160=AXIS2_PLACEMENT_3D ( 'NONE', #3102, #2975, #2055 ) ;
#3162=CYLINDRICAL_SURFACE ( 'NONE', #12756, 14.99999999999998934 ) ;
#3172=EDGE_CURVE ( 'NONE', #2573, #6716, #9218, .T. ) ;
#3177=LINE ( 'NONE', #1087, #6088 ) ;
#3184=EDGE_CURVE ( 'NONE', #8450, #8647, #11227, .T. ) ;
#3187=DIRECTION ( 'NONE',  ( -0.000000000000000000, -0.000000000000000000, -1.000000000000000000 ) ) ;
#3195=AXIS2_PLACEMENT_3D ( 'NONE', #11966, #11898, #3405 ) ;
#3196=DIRECTION ( 'NONE',  ( 0.000000000000000000, 0.000000000000000000, 1.000000000000000000 ) ) ;
#3203=EDGE_CURVE ( 'NONE', #9139, #2025, #7186, .T. ) ;
#3206=CYLINDRICAL_SURFACE ( 'NONE', #3870, 67.49999999999997158 ) ;
#3211=ORIENTED_EDGE ( 'NONE', *, *, #8678, .F. ) ;
#3213=FACE_OUTER_BOUND ( 'NONE', #12606, .T. ) ;
#3219=CARTESIAN_POINT ( 'NONE',  ( 38.99425905299097650, 101.5795188936649112, -2.500000000000004441 ) ) ;
#3240=DIRECTION ( 'NONE',  ( 1.000000000000000000, 0.000000000000000000, 0.000000000000000000 ) ) ;
#3244=CARTESIAN_POINT ( 'NONE',  ( 45.97632359910777922, 102.2167537197081657, 7.500000000000000000 ) ) ;
#3246=CIRCLE ( 'NONE', #7726, 5.000000000000004441 ) ;
#3247=ORIENTED_EDGE ( 'NONE', *, *, #3425, .F. ) ;
#3250=ORIENTED_EDGE ( 'NONE', *, *, #2581, .T. ) ;
#3251=CARTESIAN_POINT ( 'NONE',  ( -25.00000000000000355, 120.0000000000000142, -0.5000000000000000000 ) ) ;
#3252=EDGE_LOOP ( 'NONE', ( #9462, #13561, #7871, #3138, #12129, #12946, #13215, #9895 ) ) ;
#3259=DIRECTION ( 'NONE',  ( -0.000000000000000000, -0.000000000000000000, -1.000000000000000000 ) ) ;
#3261=FACE_OUTER_BOUND ( 'NONE', #1519, .T. ) ;
#3271=ORIENTED_EDGE ( 'NONE', *, *, #9104, .F. ) ;
#3275=CARTESIAN_POINT ( 'NONE',  ( -25.00000000000000355, 120.0000000000000142, 7.500000000000000000 ) ) ;
#3279=PRODUCT ( 'Soft-Touch Grip Cap Sleeve', 'Soft-Touch Grip Cap Sleeve', '', ( #6636 ) ) ;
#3287=DIRECTION ( 'NONE',  ( 0.8907235428302473501, -0.4545454545454531425, 0.000000000000000000 ) ) ;
#3292=ORIENTED_EDGE ( 'NONE', *, *, #3096, .F. ) ;
#3300=FACE_OUTER_BOUND ( 'NONE', #3599, .T. ) ;
#3314=DIRECTION ( 'NONE',  ( 1.000000000000000000, 1.850371707708595154E-15, 0.000000000000000000 ) ) ;
#3316=MANIFOLD_SOLID_BREP ( 'Cavity1', #2210 ) ;
#3321=CARTESIAN_POINT ( 'NONE',  ( 34.25812584745457201, 108.1980041606221050, -0.5000000000000000000 ) ) ;
#3322=VECTOR ( 'NONE', #8015, 1000.000000000000000 ) ;
#3323=DIRECTION ( 'NONE',  ( 1.000000000000000000, 0.000000000000000000, 0.000000000000000000 ) ) ;
#3324=DIRECTION ( 'NONE',  ( 0.000000000000000000, 0.000000000000000000, 1.000000000000000000 ) ) ;
#3326=CARTESIAN_POINT ( 'NONE',  ( 25.00000000000000355, 120.0000000000000142, -2.500000000000000000 ) ) ;
#3331=ORIENTED_EDGE ( 'NONE', *, *, #13794, .T. ) ;
#3342=TOROIDAL_SURFACE ( 'NONE', #1781, 22.99999999999999289, 2.000000000000000000 ) ;
#3346=AXIS2_PLACEMENT_3D ( 'NONE', #13034, #11044, #8801 ) ;
#3354=CARTESIAN_POINT ( 'NONE',  ( -34.40223077810360763, 107.7696006147693026, -1.740676078835883045 ) ) ;
#3357=DIRECTION ( 'NONE',  ( -0.000000000000000000, -0.000000000000000000, -1.000000000000000000 ) ) ;
#3358=CARTESIAN_POINT ( 'NONE',  ( 0.000000000000000000, 71.01020514433645303, 0.5000000000000000000 ) ) ;
#3360=AXIS2_PLACEMENT_3D ( 'NONE', #1521, #11206, #7060 ) ;
#3361=ORIENTED_EDGE ( 'NONE', *, *, #9436, .T. ) ;
#3384=CARTESIAN_POINT ( 'NONE',  ( 35.45454545454547457, 140.4866414850956460, -0.5000000000000000000 ) ) ;
#3387=CARTESIAN_POINT ( 'NONE',  ( 34.33120614476064958, 107.9646345552176001, -1.436946644489084157 ) ) ;
#3390=CARTESIAN_POINT ( 'NONE',  ( -25.00000000000000355, 120.0000000000000142, -2.499999999999998668 ) ) ;
#3391=DIRECTION ( 'NONE',  ( -0.7999999999999996003, -0.6000000000000007550, 0.000000000000000000 ) ) ;
#3405=DIRECTION ( 'NONE',  ( 1.000000000000000000, 3.495146559005123961E-15, 0.000000000000000000 ) ) ;
#3412=ADVANCED_FACE ( 'NONE', ( #10634 ), #13513, .F. ) ;
#3425=EDGE_CURVE ( 'NONE', #2956, #8890, #4272, .T. ) ;
#3430=CIRCLE ( 'NONE', #10392, 2.000000000000003109 ) ;
#3435=CARTESIAN_POINT ( 'NONE',  ( -42.16244658108819010, 105.4500712252157797, -2.499999999999998668 ) ) ;
#3440=CARTESIAN_POINT ( 'NONE',  ( -25.00000000000000355, 120.0000000000000142, 2.500000000000000000 ) ) ;
#3460=CARTESIAN_POINT ( 'NONE',  ( -40.05714107113526978, 100.9137399031062756, -2.016203456813715267 ) ) ;
#3461=CARTESIAN_POINT ( 'NONE',  ( 39.42607625790186887, 101.2633694847512658, 2.396914520158670570 ) ) ;
#3469=VERTEX_POINT ( 'NONE', #9922 ) ;
#3474=CARTESIAN_POINT ( 'NONE',  ( 40.81228451836345528, 100.6358150620708329, -0.5000000000000000000 ) ) ;
#3477=TOROIDAL_SURFACE ( 'NONE', #6410, 17.49999999999999289, 5.000000000000000000 ) ;
#3480=DIRECTION ( 'NONE',  ( 0.8907235428302473501, 0.4545454545454531425, -6.308085367188369928E-15 ) ) ;
#3481=AXIS2_PLACEMENT_3D ( 'NONE', #9716, #7600, #6625 ) ;
#3484=CARTESIAN_POINT ( 'NONE',  ( -34.27523635402735636, 108.1397967565349916, -0.9870360185550085541 ) ) ;
#3493=ORIENTED_EDGE ( 'NONE', *, *, #2852, .T. ) ;
#3498=DIRECTION ( 'NONE',  ( -0.000000000000000000, -0.000000000000000000, -1.000000000000000000 ) ) ;
#3500=CARTESIAN_POINT ( 'NONE',  ( -25.00000000000000355, 120.0000000000000142, 7.500000000000000000 ) ) ;
#3506=EDGE_CURVE ( 'NONE', #2436, #9570, #505, .T. ) ;
#3507=CARTESIAN_POINT ( 'NONE',  ( 0.000000000000000000, 71.01020514433645303, 2.500000000000000000 ) ) ;
#3508=EDGE_CURVE ( 'NONE', #11915, #9823, #3606, .T. ) ;
#3511=ORIENTED_EDGE ( 'NONE', *, *, #8678, .T. ) ;
#3519=CARTESIAN_POINT ( 'NONE',  ( 41.49999999999999289, 98.00000000000001421, 2.499999999999999556 ) ) ;
#3521=DIRECTION ( 'NONE',  ( 1.000000000000000000, 3.469446951953614978E-15, 0.000000000000000000 ) ) ;
#3525=DIRECTION ( 'NONE',  ( 0.6000000000000001998, 0.7999999999999999334, -0.000000000000000000 ) ) ;
#3526=CARTESIAN_POINT ( 'NONE',  ( -39.31542348013558552, 101.3376241895501977, -2.435478634890661631 ) ) ;
#3533=ORIENTED_EDGE ( 'NONE', *, *, #5232, .F. ) ;
#3534=CIRCLE ( 'NONE', #4672, 27.49999999999998579 ) ;
#3538=EDGE_LOOP ( 'NONE', ( #9002, #13427, #6946 ) ) ;
#3539=CARTESIAN_POINT ( 'NONE',  ( -25.00000000000000355, 120.0000000000000142, 7.500000000000000000 ) ) ;
#3551=DIRECTION ( 'NONE',  ( -1.000000000000000000, 0.000000000000000000, 0.000000000000000000 ) ) ;
#3552=CIRCLE ( 'NONE', #5352, 27.49999999999999289 ) ;
#3556=CARTESIAN_POINT ( 'NONE',  ( 42.16244658108817589, 105.4500712252157655, 7.500000000000000000 ) ) ;
#3558=CARTESIAN_POINT ( 'NONE',  ( -34.50080218526780129, 107.5336849384756164, 2.002074976903569059 ) ) ;
#3565=EDGE_CURVE ( 'NONE', #1961, #4883, #13474, .T. ) ;
#3568=CYLINDRICAL_SURFACE ( 'NONE', #13568, 79.99999999999997158 ) ;
#3571=CARTESIAN_POINT ( 'NONE',  ( -42.16244658108819010, 105.4500712252157797, 2.499999999999999556 ) ) ;
#3580=TOROIDAL_SURFACE ( 'NONE', #4252, 22.49999999999998934, 5.000000000000000000 ) ;
#3582=CARTESIAN_POINT ( 'NONE',  ( -32.50000000000000000, 110.0000000000000142, 7.500000000000000000 ) ) ;
#3591=TOROIDAL_SURFACE ( 'NONE', #245, 72.49999999999998579, 5.000000000000000000 ) ;
#3599=EDGE_LOOP ( 'NONE', ( #9568, #7347, #2129, #8200 ) ) ;
#3603=DIRECTION ( 'NONE',  ( 1.000000000000000000, 0.000000000000000000, -0.000000000000000000 ) ) ;
#3604=CARTESIAN_POINT ( 'NONE',  ( -40.79557129359547929, 100.6404192164769000, -0.7730400384045151840 ) ) ;
#3606=CIRCLE ( 'NONE', #10994, 77.49999999999998579 ) ;
#3607=CARTESIAN_POINT ( 'NONE',  ( -10.00000000000000711, 140.0000000000000000, -2.500000000000000000 ) ) ;
#3612=ORIENTED_EDGE ( 'NONE', *, *, #3506, .F. ) ;
#3613=DIRECTION ( 'NONE',  ( 0.000000000000000000, 0.000000000000000000, 1.000000000000000000 ) ) ;
#3621=CARTESIAN_POINT ( 'NONE',  ( -39.42692690461824157, 101.2627928944373963, 2.396630853396260807 ) ) ;
#3629=CYLINDRICAL_SURFACE ( 'NONE', #12358, 12.49999999999999289 ) ;
#3630=EDGE_CURVE ( 'NONE', #769, #7675, #7862, .T. ) ;
#3635=CARTESIAN_POINT ( 'NONE',  ( -34.27497211191902693, 108.1406786207261916, 0.9834270823685512530 ) ) ;
#3641=VERTEX_POINT ( 'NONE', #6980 ) ;
#3645=DIRECTION ( 'NONE',  ( 0.000000000000000000, -1.000000000000000000, 2.775557561562888984E-15 ) ) ;
#3671=ORIENTED_EDGE ( 'NONE', *, *, #11334, .T. ) ;
#3676=DIRECTION ( 'NONE',  ( 1.000000000000000000, 0.000000000000000000, 0.000000000000000000 ) ) ;
#3678=CARTESIAN_POINT ( 'NONE',  ( -39.10039359579069895, 101.4951258812516954, -2.486679384192856723 ) ) ;
#3695=CARTESIAN_POINT ( 'NONE',  ( -39.95750226049207043, 100.9609979968138589, 2.096206072712051061 ) ) ;
#3701=EDGE_CURVE ( 'NONE', #5708, #1662, #12824, .T. ) ;
#3705=CIRCLE ( 'NONE', #4602, 5.000000000000000888 ) ;
#3709=DIRECTION ( 'NONE',  ( -1.000000000000000000, 0.000000000000000000, 0.000000000000000000 ) ) ;
#3721=ORIENTED_EDGE ( 'NONE', *, *, #2749, .T. ) ;
#3745=ORIENTED_EDGE ( 'NONE', *, *, #5359, .T. ) ;
#3748=VERTEX_POINT ( 'NONE', #9494 ) ;
#3751=CARTESIAN_POINT ( 'NONE',  ( -25.00000000000000355, 120.0000000000000142, -7.500000000000000000 ) ) ;
#3754=DIRECTION ( 'NONE',  ( 0.6000000000000001998, -0.7999999999999999334, 0.000000000000000000 ) ) ;
#3757=EDGE_LOOP ( 'NONE', ( #7015, #63, #6672, #9246 ) ) ;
#3772=TOROIDAL_SURFACE ( 'NONE', #11379, 72.49999999999998579, 5.000000000000000000 ) ;
#3773=EDGE_CURVE ( 'NONE', #11361, #1587, #10115, .T. ) ;
#3775=EDGE_CURVE ( 'NONE', #12375, #7235, #1375, .T. ) ;
#3776=ADVANCED_FACE ( 'NONE', ( #1986 ), #9232, .T. ) ;
#3781=AXIS2_PLACEMENT_3D ( 'NONE', #3843, #8124, #12408 ) ;
#3791=AXIS2_PLACEMENT_3D ( 'NONE', #5276, #8304, #943 ) ;
#3793=ORIENTED_EDGE ( 'NONE', *, *, #5211, .T. ) ;
#3804=EDGE_LOOP ( 'NONE', ( #12164, #8864, #1831, #5664 ) ) ;
#3810=CARTESIAN_POINT ( 'NONE',  ( -39.06230589874905235, 109.5835921350012683, 2.499999999999999556 ) ) ;
#3814=EDGE_LOOP ( 'NONE', ( #7084, #8044, #11437, #8241, #10446, #13818, #12377, #5021, #1732, #7436, #817, #602 ) ) ;
#3823=CARTESIAN_POINT ( 'NONE',  ( -32.50000000000000000, 110.0000000000000142, 2.499999999999999556 ) ) ;
#3824=CARTESIAN_POINT ( 'NONE',  ( 37.49999999999999289, 120.0000000000000142, -2.499999999999998668 ) ) ;
#3840=CARTESIAN_POINT ( 'NONE',  ( -40.56568360645884752, 100.7114851384504135, 1.410085254968631796 ) ) ;
#3841=DIRECTION ( 'NONE',  ( 0.000000000000000000, 0.000000000000000000, 1.000000000000000000 ) ) ;
#3843=CARTESIAN_POINT ( 'NONE',  ( 35.22727272727273373, 140.0412797136805523, -2.499999999999999556 ) ) ;
#3859=ORIENTED_EDGE ( 'NONE', *, *, #3565, .T. ) ;
#3870=AXIS2_PLACEMENT_3D ( 'NONE', #909, #11625, #6306 ) ;
#3876=VERTEX_POINT ( 'NONE', #4638 ) ;
#3880=ADVANCED_FACE ( 'NONE', ( #3300 ), #8773, .T. ) ;
#3885=CARTESIAN_POINT ( 'NONE',  ( 32.95454545454546036, 135.5876619995293026, -2.499999999999998668 ) ) ;
#3887=CARTESIAN_POINT ( 'NONE',  ( 39.06230589874904524, 109.5835921350012683, -2.499999999999999556 ) ) ;
#3890=CARTESIAN_POINT ( 'NONE',  ( 35.45454545454547457, 140.4866414850956460, 2.500000000000000000 ) ) ;
#3905=DIRECTION ( 'NONE',  ( 0.000000000000000000, 0.000000000000000000, 1.000000000000000000 ) ) ;
#3910=DIRECTION ( 'NONE',  ( -0.000000000000000000, -0.000000000000000000, -1.000000000000000000 ) ) ;
#3914=ORIENTED_EDGE ( 'NONE', *, *, #2830, .T. ) ;
#3934=CARTESIAN_POINT ( 'NONE',  ( -25.00000000000000355, 120.0000000000000142, 2.500000000000000000 ) ) ;
#3951=CARTESIAN_POINT ( 'NONE',  ( -34.25812584745457201, 108.1980041606221192, 0.5000000000000000000 ) ) ;
#3955=EDGE_CURVE ( 'NONE', #3876, #7882, #8922, .T. ) ;
#3960=DIRECTION ( 'NONE',  ( 0.000000000000000000, -1.000000000000000000, 0.000000000000000000 ) ) ;
#3971=VERTEX_POINT ( 'NONE', #4562 ) ;
#3981=ORIENTED_EDGE ( 'NONE', *, *, #9436, .F. ) ;
#3983=DIRECTION ( 'NONE',  ( 1.000000000000000000, 0.000000000000000000, 0.000000000000000000 ) ) ;
#3985=CARTESIAN_POINT ( 'NONE',  ( 31.81818181818183433, 133.3608531424536920, -0.5000000000000000000 ) ) ;
#3993=ORIENTED_EDGE ( 'NONE', *, *, #5211, .F. ) ;
#3998=DIRECTION ( 'NONE',  ( 0.000000000000000000, 0.000000000000000000, 1.000000000000000000 ) ) ;
#4029=CARTESIAN_POINT ( 'NONE',  ( 25.00000000000000355, 120.0000000000000142, -0.5000000000000000000 ) ) ;
#4032=AXIS2_PLACEMENT_3D ( 'NONE', #8253, #6857, #2793 ) ;
#4037=LINE ( 'NONE', #8320, #6199 ) ;
#4044=AXIS2_PLACEMENT_3D ( 'NONE', #7399, #6227, #6159 ) ;
#4047=LINE ( 'NONE', #13632, #5798 ) ;
#4050=EDGE_CURVE ( 'NONE', #13751, #5579, #10182, .T. ) ;
#4061=AXIS2_PLACEMENT_3D ( 'NONE', #4660, #8947, #6838 ) ;
#4063=EDGE_CURVE ( 'NONE', #7235, #9684, #10043, .T. ) ;
#4077=ORIENTED_EDGE ( 'NONE', *, *, #2119, .T. ) ;
#4080=CARTESIAN_POINT ( 'NONE',  ( -40.81228451836347659, 100.6358150620708471, 0.000000000000000000 ) ) ;
#4085=DIRECTION ( 'NONE',  ( 1.000000000000000000, 0.000000000000000000, 0.000000000000000000 ) ) ;
#4092=ORIENTED_EDGE ( 'NONE', *, *, #9830, .T. ) ;
#4095=LINE ( 'NONE', #4162, #9403 ) ;
#4108=CARTESIAN_POINT ( 'NONE',  ( -35.06230589874904524, 106.5835921350012825, -2.486789939184904430 ) ) ;
#4111=TOROIDAL_SURFACE ( 'NONE', #5445, 22.49999999999998934, 5.000000000000000000 ) ;
#4131=EDGE_LOOP ( 'NONE', ( #2333, #10811, #2091, #3793 ) ) ;
#4140=CARTESIAN_POINT ( 'NONE',  ( 39.06230589874904524, 109.5835921350012683, 2.499999999999999556 ) ) ;
#4161=LINE ( 'NONE', #2061, #2513 ) ;
#4162=CARTESIAN_POINT ( 'NONE',  ( 30.68181818181819054, 131.1340442853780530, 7.500000000000000000 ) ) ;
#4202=DIRECTION ( 'NONE',  ( -0.6000000000000001998, -0.7999999999999998224, 0.000000000000000000 ) ) ;
#4206=ADVANCED_FACE ( 'NONE', ( #2961 ), #8549, .T. ) ;
#4214=VERTEX_POINT ( 'NONE', #10588 ) ;
#4217=DIRECTION ( 'NONE',  ( 0.000000000000000000, -1.000000000000000000, 0.000000000000000000 ) ) ;
#4224=CARTESIAN_POINT ( 'NONE',  ( -30.68181818181819054, 131.1340442853780814, -2.499999999999998668 ) ) ;
#4230=DIRECTION ( 'NONE',  ( 1.000000000000000000, 0.000000000000000000, 0.000000000000000000 ) ) ;
#4231=CIRCLE ( 'NONE', #7728, 12.49999999999999289 ) ;
#4234=LINE ( 'NONE', #9509, #2798 ) ;
#4242=CARTESIAN_POINT ( 'NONE',  ( -25.00000000000000355, 120.0000000000000142, -0.5000000000000000000 ) ) ;
#4251=AXIS2_PLACEMENT_3D ( 'NONE', #1098, #5357, #9648 ) ;
#4252=AXIS2_PLACEMENT_3D ( 'NONE', #668, #11182, #467 ) ;
#4261=AXIS2_PLACEMENT_3D ( 'NONE', #1861, #5089, #821 ) ;
#4265=EDGE_LOOP ( 'NONE', ( #6517, #4426, #637, #6324 ) ) ;
#4272=CIRCLE ( 'NONE', #6522, 27.49999999999998579 ) ;
#4275=CIRCLE ( 'NONE', #497, 4.999999999999996447 ) ;
#4277=DIRECTION ( 'NONE',  ( 0.000000000000000000, 0.000000000000000000, 1.000000000000000000 ) ) ;
#4290=DIRECTION ( 'NONE',  ( -0.000000000000000000, -0.000000000000000000, -1.000000000000000000 ) ) ;
#4293=CARTESIAN_POINT ( 'NONE',  ( 25.00000000000000355, 120.0000000000000142, 2.499999999999999556 ) ) ;
#4298=DIRECTION ( 'NONE',  ( 1.000000000000000000, -1.110223024625156935E-15, 0.000000000000000000 ) ) ;
#4300=ORIENTED_EDGE ( 'NONE', *, *, #6429, .F. ) ;
#4308=ADVANCED_FACE ( 'NONE', ( #9955 ), #3772, .T. ) ;
#4317=AXIS2_PLACEMENT_3D ( 'NONE', #4140, #6387, #1132 ) ;
#4321=DIRECTION ( 'NONE',  ( -0.5999999999999989786, -0.8000000000000008216, 0.000000000000000000 ) ) ;
#4330=CIRCLE ( 'NONE', #9943, 24.99999999999998934 ) ;
#4331=PLANE ( 'NONE',  #5327 ) ;
#4333=CARTESIAN_POINT ( 'NONE',  ( -42.16244658108818300, 105.4500712252157655, 2.500000000000000000 ) ) ;
#4339=ORIENTED_EDGE ( 'NONE', *, *, #9198, .T. ) ;
#4343=TOROIDAL_SURFACE ( 'NONE', #12464, 16.99999999999998934, 2.000000000000000000 ) ;
#4344=DIRECTION ( 'NONE',  ( 0.5952233065713573579, -0.8035603370713738647, 0.000000000000000000 ) ) ;
#4355=LINE ( 'NONE', #5543, #11669 ) ;
#4357=CARTESIAN_POINT ( 'NONE',  ( -35.20000000000000995, 106.3999999999999915, 0.5000000000000000000 ) ) ;
#4363=ADVANCED_FACE ( 'NONE', ( #6580 ), #4331, .T. ) ;
#4367=DIRECTION ( 'NONE',  ( 1.000000000000000000, 0.000000000000000000, 0.000000000000000000 ) ) ;
#4378=CIRCLE ( 'NONE', #10436, 27.49999999999999289 ) ;
#4381=AXIS2_PLACEMENT_3D ( 'NONE', #826, #10154, #6081 ) ;
#4388=CARTESIAN_POINT ( 'NONE',  ( -32.50000000000000000, 110.0000000000000142, 2.500000000000000000 ) ) ;
#4390=CARTESIAN_POINT ( 'NONE',  ( 39.06230589874905235, 109.5835921350012683, -2.499999999999999556 ) ) ;
#4401=DIRECTION ( 'NONE',  ( 0.6000000000000001998, 0.7999999999999999334, 0.000000000000000000 ) ) ;
#4402=CARTESIAN_POINT ( 'NONE',  ( -34.46489414126432393, 107.6161901685304514, -1.920132901535060777 ) ) ;
#4404=FACE_OUTER_BOUND ( 'NONE', #8429, .T. ) ;
#4410=CARTESIAN_POINT ( 'NONE',  ( -39.06230589874905235, 109.5835921350012683, 2.499999999999999556 ) ) ;
#4415=CARTESIAN_POINT ( 'NONE',  ( 38.16244658108818300, 102.4500712252157655, -2.500000000000000444 ) ) ;
#4421=DIRECTION ( 'NONE',  ( -0.8000000000000008216, 0.5999999999999988676, 0.000000000000000000 ) ) ;
#4426=ORIENTED_EDGE ( 'NONE', *, *, #10142, .T. ) ;
#4427=CARTESIAN_POINT ( 'NONE',  ( -52.50000000000000000, 120.0000000000000142, -2.499999999999998668 ) ) ;
#4428=DIRECTION ( 'NONE',  ( -0.000000000000000000, -0.000000000000000000, -1.000000000000000000 ) ) ;
#4430=ORIENTED_EDGE ( 'NONE', *, *, #480, .F. ) ;
#4431=DIRECTION ( 'NONE',  ( -0.000000000000000000, -0.000000000000000000, -1.000000000000000000 ) ) ;
#4439=DIRECTION ( 'NONE',  ( -0.6000000000000001998, 0.7999999999999999334, 0.000000000000000000 ) ) ;
#4448=FACE_OUTER_BOUND ( 'NONE', #1707, .T. ) ;
#4452=ADVANCED_FACE ( 'NONE', ( #6930 ), #1610, .T. ) ;
#4466=VERTEX_POINT ( 'NONE', #7005 ) ;
#4469=EDGE_LOOP ( 'NONE', ( #1325, #9795, #13468, #9680 ) ) ;
#4488=CARTESIAN_POINT ( 'NONE',  ( 25.00000000000000355, 120.0000000000000142, 0.5000000000000000000 ) ) ;
#4501=ORIENTED_EDGE ( 'NONE', *, *, #11606, .T. ) ;
#4512=FACE_OUTER_BOUND ( 'NONE', #2066, .T. ) ;
#4516=ORIENTED_EDGE ( 'NONE', *, *, #8243, .T. ) ;
#4550=ORIENTED_EDGE ( 'NONE', *, *, #7059, .T. ) ;
#4552=CIRCLE ( 'NONE', #6590, 77.99999999999997158 ) ;
#4560=EDGE_CURVE ( 'NONE', #5087, #3748, #11616, .T. ) ;
#4562=CARTESIAN_POINT ( 'NONE',  ( 38.89115197531749857, 101.6687180808697377, 2.499999999999999556 ) ) ;
#4575=VERTEX_POINT ( 'NONE', #3985 ) ;
#4586=CARTESIAN_POINT ( 'NONE',  ( -38.99475364604207073, 101.5790910151996655, -2.500000000000037748 ) ) ;
#4589=CARTESIAN_POINT ( 'NONE',  ( 38.99475364604206362, 101.5790910151996655, 2.500000000000036859 ) ) ;
#4598=ORIENTED_EDGE ( 'NONE', *, *, #13517, .F. ) ;
#4601=EDGE_LOOP ( 'NONE', ( #11008, #7257, #9917, #2629 ) ) ;
#4602=AXIS2_PLACEMENT_3D ( 'NONE', #3810, #4935, #8163 ) ;
#4604=CARTESIAN_POINT ( 'NONE',  ( -38.99425905299099071, 101.5795188936649254, 2.500000000000002665 ) ) ;
#4606=VECTOR ( 'NONE', #13610, 1000.000000000000000 ) ;
#4611=VERTEX_POINT ( 'NONE', #9324 ) ;
#4613=CIRCLE ( 'NONE', #13394, 2.000000000000003997 ) ;
#4616=ORIENTED_EDGE ( 'NONE', *, *, #10569, .T. ) ;
#4617=DIRECTION ( 'NONE',  ( 0.000000000000000000, 1.000000000000000000, 0.000000000000000000 ) ) ;
#4623=CARTESIAN_POINT ( 'NONE',  ( -34.46489652880495669, 107.6161854625081844, 1.920135329999819174 ) ) ;
#4631=ORIENTED_EDGE ( 'NONE', *, *, #13240, .T. ) ;
#4638=CARTESIAN_POINT ( 'NONE',  ( 37.50000000000002132, 144.4948974278317735, 2.499999999999999556 ) ) ;
#4642=VECTOR ( 'NONE', #4202, 999.9999999999998863 ) ;
#4643=DIRECTION ( 'NONE',  ( 1.000000000000000000, 0.000000000000000000, 0.000000000000000000 ) ) ;
#4659=DIRECTION ( 'NONE',  ( 1.000000000000000000, 3.558407130208836623E-15, 0.000000000000000000 ) ) ;
#4660=CARTESIAN_POINT ( 'NONE',  ( -25.00000000000000355, 120.0000000000000142, 0.5000000000000000000 ) ) ;
#4663=DIRECTION ( 'NONE',  ( 1.000000000000000000, 0.000000000000000000, 0.000000000000000000 ) ) ;
#4664=ADVANCED_FACE ( 'NONE', ( #140 ), #13194, .T. ) ;
#4672=AXIS2_PLACEMENT_3D ( 'NONE', #11967, #6642, #13047 ) ;
#4679=CARTESIAN_POINT ( 'NONE',  ( -39.75092559767095679, 101.0685047868946072, 2.236846530894073926 ) ) ;
#4692=DIRECTION ( 'NONE',  ( 0.000000000000000000, 0.000000000000000000, 1.000000000000000000 ) ) ;
#4696=AXIS2_PLACEMENT_3D ( 'NONE', #2117, #3960, #8502 ) ;
#4704=EDGE_LOOP ( 'NONE', ( #8540, #6910, #4550, #6702, #1812 ) ) ;
#4708=DIRECTION ( 'NONE',  ( 0.000000000000000000, 1.000000000000000000, 0.000000000000000000 ) ) ;
#4711=DIRECTION ( 'NONE',  ( 1.387778780781444492E-15, 1.000000000000000000, -1.734723475976805615E-16 ) ) ;
#4712=PRODUCT_DEFINITION ( 'UNKNOWN', '', #8199, #5888 ) ;
#4714=CIRCLE ( 'NONE', #4251, 82.49999999999998579 ) ;
#4722=VERTEX_POINT ( 'NONE', #1111 ) ;
#4728=VECTOR ( 'NONE', #429, 1000.000000000000000 ) ;
#4732=ORIENTED_EDGE ( 'NONE', *, *, #10645, .F. ) ;
#4733=FACE_OUTER_BOUND ( 'NONE', #3034, .T. ) ;
#4751=CARTESIAN_POINT ( 'NONE',  ( 25.00000000000000355, 120.0000000000000142, 2.500000000000000000 ) ) ;
#4752=ADVANCED_FACE ( 'NONE', ( #10980 ), #1492, .F. ) ;
#4773=DIRECTION ( 'NONE',  ( 1.000000000000000000, 0.000000000000000000, 0.000000000000000000 ) ) ;
#4776=ORIENTED_EDGE ( 'NONE', *, *, #4050, .F. ) ;
#4777=CIRCLE ( 'NONE', #8797, 4.999999999999998224 ) ;
#4786=DIRECTION ( 'NONE',  ( 1.000000000000000000, 0.000000000000000000, 0.000000000000000000 ) ) ;
#4791=CARTESIAN_POINT ( 'NONE',  ( 41.99999999999999289, 120.0000000000000142, 2.500000000000000000 ) ) ;
#4800=CIRCLE ( 'NONE', #5675, 16.99999999999998934 ) ;
#4810=DIRECTION ( 'NONE',  ( -0.000000000000000000, -0.000000000000000000, -1.000000000000000000 ) ) ;
#4812=FACE_OUTER_BOUND ( 'NONE', #13187, .T. ) ;
#4821=EDGE_CURVE ( 'NONE', #3641, #5368, #13675, .T. ) ;
#4822=AXIS2_PLACEMENT_3D ( 'NONE', #12018, #9710, #8653 ) ;
#4828=SHAPE_DEFINITION_REPRESENTATION ( #13178, #5134 ) ;
#4831=CYLINDRICAL_SURFACE ( 'NONE', #13158, 4.999999999999997335 ) ;
#4833=FACE_OUTER_BOUND ( 'NONE', #2920, .T. ) ;
#4835=ADVANCED_FACE ( 'NONE', ( #13276 ), #4831, .T. ) ;
#4837=ORIENTED_EDGE ( 'NONE', *, *, #1540, .T. ) ;
#4859=DIRECTION ( 'NONE',  ( -0.8000000000000000444, 0.5999999999999999778, 0.000000000000000000 ) ) ;
#4868=DIRECTION ( 'NONE',  ( 1.000000000000000000, 0.000000000000000000, 0.000000000000000000 ) ) ;
#4876=DIRECTION ( 'NONE',  ( 1.000000000000000000, 0.000000000000000000, 0.000000000000000000 ) ) ;
#4883=VERTEX_POINT ( 'NONE', #4108 ) ;
#4884=DIRECTION ( 'NONE',  ( -0.7999999999999977129, -0.6000000000000030864, 0.000000000000000000 ) ) ;
#4901=AXIS2_PLACEMENT_3D ( 'NONE', #9790, #8725, #6564 ) ;
#4906=CARTESIAN_POINT ( 'NONE',  ( -34.63132358390376453, 107.2645221665701456, 2.217002873864903911 ) ) ;
#4910=ORIENTED_EDGE ( 'NONE', *, *, #6885, .T. ) ;
#4935=DIRECTION ( 'NONE',  ( 0.5952233065713573579, -0.8035603370713738647, 3.056366244416776485E-15 ) ) ;
#4938=ORIENTED_EDGE ( 'NONE', *, *, #8857, .T. ) ;
#4939=CARTESIAN_POINT ( 'NONE',  ( 25.00000000000000355, 120.0000000000000142, -0.5000000000000000000 ) ) ;
#4945=DIRECTION ( 'NONE',  ( 0.000000000000000000, 0.000000000000000000, -1.000000000000000000 ) ) ;
#4947=CARTESIAN_POINT ( 'NONE',  ( -35.06230589874905235, 106.5835921350012825, 7.500000000000000000 ) ) ;
#4957=FACE_OUTER_BOUND ( 'NONE', #1499, .T. ) ;
#4958=DIRECTION ( 'NONE',  ( -0.000000000000000000, -0.000000000000000000, -1.000000000000000000 ) ) ;
#4968=ORIENTED_EDGE ( 'NONE', *, *, #3203, .F. ) ;
#4980=EDGE_CURVE ( 'NONE', #8180, #780, #11571, .T. ) ;
#4989=FACE_OUTER_BOUND ( 'NONE', #9534, .T. ) ;
#4992=DIRECTION ( 'NONE',  ( 1.000000000000000000, 0.000000000000000000, 0.000000000000000000 ) ) ;
#5003=ADVANCED_FACE ( 'NONE', ( #4512 ), #6424, .T. ) ;
#5005=CIRCLE ( 'NONE', #11712, 4.999999999999997335 ) ;
#5021=ORIENTED_EDGE ( 'NONE', *, *, #5865, .F. ) ;
#5022=ORIENTED_EDGE ( 'NONE', *, *, #12971, .T. ) ;
#5024=CARTESIAN_POINT ( 'NONE',  ( 39.06230589874905235, 109.5835921350012825, -2.499999999999999556 ) ) ;
#5031=CIRCLE ( 'NONE', #6587, 2.000000000000003109 ) ;
#5036=ORIENTED_EDGE ( 'NONE', *, *, #1750, .F. ) ;
#5047=APPLICATION_CONTEXT ( 'automotive_design' ) ;
#5053=AXIS2_PLACEMENT_3D ( 'NONE', #1908, #7302, #5197 ) ;
#5058=ORIENTED_EDGE ( 'NONE', *, *, #5095, .F. ) ;
#5060=EDGE_CURVE ( 'NONE', #12157, #11361, #13414, .T. ) ;
#5070=EDGE_CURVE ( 'NONE', #8647, #6878, #623, .T. ) ;
#5079=ADVANCED_FACE ( 'NONE', ( #2279 ), #10819, .T. ) ;
#5083=DIRECTION ( 'NONE',  ( 0.000000000000000000, 1.000000000000000000, 0.000000000000000000 ) ) ;
#5087=VERTEX_POINT ( 'NONE', #12247 ) ;
#5089=DIRECTION ( 'NONE',  ( 0.000000000000000000, 0.000000000000000000, 1.000000000000000000 ) ) ;
#5093=CARTESIAN_POINT ( 'NONE',  ( 0.000000000000000000, 71.01020514433645303, 2.500000000000000000 ) ) ;
#5095=EDGE_CURVE ( 'NONE', #1278, #5338, #55, .T. ) ;
#5110=DIRECTION ( 'NONE',  ( -0.000000000000000000, -0.000000000000000000, -1.000000000000000000 ) ) ;
#5111=AXIS2_PLACEMENT_3D ( 'NONE', #3556, #5896, #3709 ) ;
#5112=ORIENTED_EDGE ( 'NONE', *, *, #8243, .F. ) ;
#5119=DIRECTION ( 'NONE',  ( 0.000000000000000000, 1.000000000000000000, 1.734723475976805615E-16 ) ) ;
#5130=EDGE_LOOP ( 'NONE', ( #1352, #6047, #8763, #10175 ) ) ;
#5132=EDGE_LOOP ( 'NONE', ( #13795, #11373, #1072, #4300 ) ) ;
#5134=SHAPE_REPRESENTATION ( 'Soft-Touch Grip Cap Sleeve', ( #8193 ), #1690 ) ;
#5136=ORIENTED_EDGE ( 'NONE', *, *, #8223, .F. ) ;
#5142=DIRECTION ( 'NONE',  ( -0.000000000000000000, -0.000000000000000000, -1.000000000000000000 ) ) ;
#5143=CIRCLE ( 'NONE', #7819, 14.99999999999998934 ) ;
#5148=ORIENTED_EDGE ( 'NONE', *, *, #8413, .F. ) ;
#5152=ADVANCED_FACE ( 'NONE', ( #7810 ), #550, .T. ) ;
#5158=CARTESIAN_POINT ( 'NONE',  ( 25.00000000000000355, 120.0000000000000142, 2.500000000000000000 ) ) ;
#5160=DIRECTION ( 'NONE',  ( 1.000000000000000000, 0.000000000000000000, 0.000000000000000000 ) ) ;
#5166=CARTESIAN_POINT ( 'NONE',  ( 25.00000000000000355, 120.0000000000000142, -2.499999999999998668 ) ) ;
#5168=DIRECTION ( 'NONE',  ( 0.6466635011015220424, 0.7627754036039191554, 8.974258851345311771E-16 ) ) ;
#5170=ADVANCED_FACE ( 'NONE', ( #1436 ), #3070, .F. ) ;
#5185=DIRECTION ( 'NONE',  ( 0.000000000000000000, 0.000000000000000000, 1.000000000000000000 ) ) ;
#5190=CIRCLE ( 'NONE', #8764, 14.99999999999998934 ) ;
#5197=DIRECTION ( 'NONE',  ( -0.5999999999999989786, 0.8000000000000008216, 0.000000000000000000 ) ) ;
#5199=ORIENTED_EDGE ( 'NONE', *, *, #3184, .F. ) ;
#5200=ORIENTED_EDGE ( 'NONE', *, *, #12273, .T. ) ;
#5211=EDGE_CURVE ( 'NONE', #10135, #4575, #5531, .T. ) ;
#5231=DIRECTION ( 'NONE',  ( 0.7627754036039191554, -0.6466635011015219314, 8.673617379884041389E-16 ) ) ;
#5232=EDGE_CURVE ( 'NONE', #10350, #9880, #11325, .T. ) ;
#5239=LINE ( 'NONE', #12629, #3014 ) ;
#5247=EDGE_CURVE ( 'NONE', #11915, #13399, #13333, .T. ) ;
#5250=AXIS2_PLACEMENT_3D ( 'NONE', #2988, #6419, #6285 ) ;
#5254=AXIS2_PLACEMENT_3D ( 'NONE', #13754, #12950, #10682 ) ;
#5259=CARTESIAN_POINT ( 'NONE',  ( -34.73643445648811934, 107.0738672501280604, -2.329477027598934491 ) ) ;
#5264=ORIENTED_EDGE ( 'NONE', *, *, #11606, .F. ) ;
#5265=EDGE_CURVE ( 'NONE', #7235, #8382, #2538, .T. ) ;
#5276=CARTESIAN_POINT ( 'NONE',  ( 25.00000000000000355, 120.0000000000000142, 0.5000000000000000000 ) ) ;
#5280=CIRCLE ( 'NONE', #7486, 22.99999999999999645 ) ;
#5285=AXIS2_PLACEMENT_3D ( 'NONE', #4333, #12853, #9814 ) ;
#5292=FACE_OUTER_BOUND ( 'NONE', #1200, .T. ) ;
#5294=AXIS2_PLACEMENT_3D ( 'NONE', #630, #1451, #6998 ) ;
#5307=DIRECTION ( 'NONE',  ( 0.000000000000000000, 0.000000000000000000, 1.000000000000000000 ) ) ;
#5309=AXIS2_PLACEMENT_3D ( 'NONE', #10207, #615, #676 ) ;
#5314=ORIENTED_EDGE ( 'NONE', *, *, #1669, .F. ) ;
#5321=ORIENTED_EDGE ( 'NONE', *, *, #3172, .T. ) ;
#5327=AXIS2_PLACEMENT_3D ( 'NONE', #2165, #10713, #4401 ) ;
#5328=CARTESIAN_POINT ( 'NONE',  ( -34.63116476221792794, 107.2647840444379312, -2.216888271186469250 ) ) ;
#5337=DIRECTION ( 'NONE',  ( 0.8035603370713739757, 0.5952233065713573579, 0.000000000000000000 ) ) ;
#5338=VERTEX_POINT ( 'NONE', #1196 ) ;
#5339=FACE_OUTER_BOUND ( 'NONE', #4265, .T. ) ;
#5342=DIRECTION ( 'NONE',  ( -0.000000000000000000, -0.000000000000000000, -1.000000000000000000 ) ) ;
#5346=FACE_OUTER_BOUND ( 'NONE', #379, .T. ) ;
#5352=AXIS2_PLACEMENT_3D ( 'NONE', #10792, #8765, #1203 ) ;
#5354=CARTESIAN_POINT ( 'NONE',  ( -37.50000000000002132, 144.4948974278317735, -2.499999999999998668 ) ) ;
#5357=DIRECTION ( 'NONE',  ( -0.000000000000000000, -0.000000000000000000, -1.000000000000000000 ) ) ;
#5359=EDGE_CURVE ( 'NONE', #3971, #8890, #5005, .T. ) ;
#5365=AXIS2_PLACEMENT_3D ( 'NONE', #7424, #3998, #3081 ) ;
#5368=VERTEX_POINT ( 'NONE', #8758 ) ;
#5379=VERTEX_POINT ( 'NONE', #2523 ) ;
#5380=CIRCLE ( 'NONE', #4261, 14.99999999999998934 ) ;
#5384=DIRECTION ( 'NONE',  ( -0.4545454545454531425, 0.8907235428302472391, 0.000000000000000000 ) ) ;
#5388=CARTESIAN_POINT ( 'NONE',  ( 40.05868326948369429, 100.9130297721161043, -2.014878269406404687 ) ) ;
#5392=AXIS2_PLACEMENT_3D ( 'NONE', #10676, #11537, #11800 ) ;
#5414=ORIENTED_EDGE ( 'NONE', *, *, #2310, .T. ) ;
#5420=CARTESIAN_POINT ( 'NONE',  ( -25.00000000000000355, 120.0000000000000142, -2.500000000000000000 ) ) ;
#5424=DIRECTION ( 'NONE',  ( 0.000000000000000000, 0.000000000000000000, 1.000000000000000000 ) ) ;
#5428=CARTESIAN_POINT ( 'NONE',  ( 40.34010237645983921, 100.7894366958197594, 1.747896926826554731 ) ) ;
#5432=VECTOR ( 'NONE', #6493, 1000.000000000000000 ) ;
#5436=AXIS2_PLACEMENT_3D ( 'NONE', #6315, #12775, #9342 ) ;
#5443=DIRECTION ( 'NONE',  ( -0.000000000000000000, -0.000000000000000000, -1.000000000000000000 ) ) ;
#5445=AXIS2_PLACEMENT_3D ( 'NONE', #5762, #13150, #4786 ) ;
#5458=CARTESIAN_POINT ( 'NONE',  ( -34.58461996471805122, 107.3565440455617903, -2.151643583074648536 ) ) ;
#5459=CARTESIAN_POINT ( 'NONE',  ( 42.16244658108818300, 105.4500712252157655, 2.499999999999999556 ) ) ;
#5463=VERTEX_POINT ( 'NONE', #6726 ) ;
#5465=CIRCLE ( 'NONE', #7946, 77.99999999999997158 ) ;
#5470=DIRECTION ( 'NONE',  ( 1.000000000000000000, 0.000000000000000000, 0.000000000000000000 ) ) ;
#5491=CARTESIAN_POINT ( 'NONE',  ( 25.00000000000000355, 120.0000000000000142, -0.5000000000000000000 ) ) ;
#5493=DIRECTION ( 'NONE',  ( -1.000000000000000000, 0.000000000000000000, 0.000000000000000000 ) ) ;
#5498=ADVANCED_FACE ( 'NONE', ( #9396 ), #3206, .F. ) ;
#5499=CARTESIAN_POINT ( 'NONE',  ( 25.00000000000000355, 120.0000000000000142, -0.5000000000000000000 ) ) ;
#5502=DIRECTION ( 'NONE',  ( -0.000000000000000000, -0.000000000000000000, -1.000000000000000000 ) ) ;
#5506=CARTESIAN_POINT ( 'NONE',  ( 25.00000000000000355, 120.0000000000000142, -7.500000000000000000 ) ) ;
#5509=ORIENTED_EDGE ( 'NONE', *, *, #13517, .T. ) ;
#5510=ORIENTED_EDGE ( 'NONE', *, *, #5359, .F. ) ;
#5521=ORIENTED_EDGE ( 'NONE', *, *, #13254, .T. ) ;
#5531=CIRCLE ( 'NONE', #5309, 69.99999999999998579 ) ;
#5537=DIRECTION ( 'NONE',  ( 0.6466635011015214873, -0.7627754036039198215, 3.014552924381575957E-15 ) ) ;
#5543=CARTESIAN_POINT ( 'NONE',  ( 10.99999999999999289, 147.0000000000000284, 7.500000000000000000 ) ) ;
#5557=VECTOR ( 'NONE', #1036, 1000.000000000000000 ) ;
#5565=EDGE_CURVE ( 'NONE', #2097, #11234, #1402, .T. ) ;
#5570=AXIS2_PLACEMENT_3D ( 'NONE', #2384, #2319, #6598 ) ;
#5579=VERTEX_POINT ( 'NONE', #3474 ) ;
#5585=CARTESIAN_POINT ( 'NONE',  ( 45.97632359910777922, 102.2167537197081657, 2.499999999999999556 ) ) ;
#5590=CARTESIAN_POINT ( 'NONE',  ( 35.04450421339217314, 112.5597086678580609, 7.500000000000000000 ) ) ;
#5591=CIRCLE ( 'NONE', #13494, 4.999999999999997335 ) ;
#5602=AXIS2_PLACEMENT_3D ( 'NONE', #12805, #5083, #6338 ) ;
#5605=ORIENTED_EDGE ( 'NONE', *, *, #13221, .T. ) ;
#5606=AXIS2_PLACEMENT_3D ( 'NONE', #2701, #10339, #6975 ) ;
#5612=AXIS2_PLACEMENT_3D ( 'NONE', #1216, #13009, #12003 ) ;
#5613=CARTESIAN_POINT ( 'NONE',  ( -37.50000000000002132, 144.4948974278317735, 2.499999999999999556 ) ) ;
#5621=FACE_OUTER_BOUND ( 'NONE', #1058, .T. ) ;
#5623=CARTESIAN_POINT ( 'NONE',  ( -25.00000000000000355, 120.0000000000000142, -7.500000000000000000 ) ) ;
#5632=VERTEX_POINT ( 'NONE', #12910 ) ;
#5651=EDGE_CURVE ( 'NONE', #214, #863, #6124, .T. ) ;
#5656=DIRECTION ( 'NONE',  ( -0.6000000000000001998, -0.7999999999999998224, 0.000000000000000000 ) ) ;
#5657=CARTESIAN_POINT ( 'NONE',  ( -40.05868326948371561, 100.9130297721161327, 2.014878269406402467 ) ) ;
#5660=ADVANCED_FACE ( 'NONE', ( #10700 ), #6507, .T. ) ;
#5664=ORIENTED_EDGE ( 'NONE', *, *, #12704, .F. ) ;
#5666=EDGE_CURVE ( 'NONE', #6479, #9684, #13082, .T. ) ;
#5675=AXIS2_PLACEMENT_3D ( 'NONE', #3440, #10802, #40 ) ;
#5677=EDGE_CURVE ( 'NONE', #2194, #2762, #7443, .T. ) ;
#5678=CARTESIAN_POINT ( 'NONE',  ( -34.40224804986665674, 107.7695571918731758, 1.740729949763268447 ) ) ;
#5682=ORIENTED_EDGE ( 'NONE', *, *, #8070, .F. ) ;
#5684=DIRECTION ( 'NONE',  ( -0.000000000000000000, -0.000000000000000000, -1.000000000000000000 ) ) ;
#5705=CIRCLE ( 'NONE', #5954, 71.99999999999998579 ) ;
#5707=CYLINDRICAL_SURFACE ( 'NONE', #11310, 27.49999999999998934 ) ;
#5708=VERTEX_POINT ( 'NONE', #12118 ) ;
#5715=CARTESIAN_POINT ( 'NONE',  ( 32.72727272727274084, 135.1423002281141805, 2.500000000000000000 ) ) ;
#5718=AXIS2_PLACEMENT_3D ( 'NONE', #9144, #13466, #13395 ) ;
#5722=ADVANCED_BREP_SHAPE_REPRESENTATION ( '', ( #3316, #8193 ), #1690 ) ;
#5725=CARTESIAN_POINT ( 'NONE',  ( -31.81818181818181657, 133.3608531424536920, -0.5000000000000000000 ) ) ;
#5737=CIRCLE ( 'NONE', #11122, 22.99999999999999645 ) ;
#5738=CARTESIAN_POINT ( 'NONE',  ( -25.00000000000000355, 120.0000000000000142, 7.500000000000000000 ) ) ;
#5743=DIRECTION ( 'NONE',  ( 0.000000000000000000, 0.000000000000000000, 1.000000000000000000 ) ) ;
#5748=EDGE_CURVE ( 'NONE', #1913, #2762, #2770, .T. ) ;
#5750=EDGE_CURVE ( 'NONE', #8935, #624, #4777, .T. ) ;
#5759=ORIENTED_EDGE ( 'NONE', *, *, #4560, .F. ) ;
#5762=CARTESIAN_POINT ( 'NONE',  ( 25.00000000000000355, 120.0000000000000142, -2.499999999999998668 ) ) ;
#5774=ORIENTED_EDGE ( 'NONE', *, *, #9875, .T. ) ;
#5788=CARTESIAN_POINT ( 'NONE',  ( -39.74871155318043492, 101.0697170996391492, -2.238193420436155989 ) ) ;
#5795=CARTESIAN_POINT ( 'NONE',  ( -39.06230589874905945, 109.5835921350012825, 7.500000000000000000 ) ) ;
#5798=VECTOR ( 'NONE', #8330, 999.9999999999998863 ) ;
#5812=DIRECTION ( 'NONE',  ( 0.000000000000000000, 0.000000000000000000, 1.000000000000000000 ) ) ;
#5818=VECTOR ( 'NONE', #9575, 999.9999999999998863 ) ;
#5820=DIRECTION ( 'NONE',  ( 1.000000000000000000, 0.000000000000000000, 0.000000000000000000 ) ) ;
#5824=EDGE_LOOP ( 'NONE', ( #1022, #4339, #6110, #2954 ) ) ;
#5833=ORIENTED_EDGE ( 'NONE', *, *, #9547, .T. ) ;
#5837=AXIS2_PLACEMENT_3D ( 'NONE', #12779, #12581, #8354 ) ;
#5852=ORIENTED_EDGE ( 'NONE', *, *, #1750, .T. ) ;
#5865=EDGE_CURVE ( 'NONE', #7422, #5463, #6126, .T. ) ;
#5867=DIRECTION ( 'NONE',  ( 0.8907235428302465730, 0.4545454545454549189, -0.000000000000000000 ) ) ;
#5868=EDGE_CURVE ( 'NONE', #11234, #8040, #7664, .T. ) ;
#5871=CARTESIAN_POINT ( 'NONE',  ( -42.16244658108818300, 105.4500712252157797, 7.500000000000000000 ) ) ;
#5879=ORIENTED_EDGE ( 'NONE', *, *, #11334, .F. ) ;
#5887=DIRECTION ( 'NONE',  ( 1.000000000000000000, 0.000000000000000000, 0.000000000000000000 ) ) ;
#5888=PRODUCT_DEFINITION_CONTEXT ( 'detailed design', #9879, 'design' ) ;
#5896=DIRECTION ( 'NONE',  ( -0.000000000000000000, -0.000000000000000000, -1.000000000000000000 ) ) ;
#5937=CARTESIAN_POINT ( 'NONE',  ( -40.34010237645985342, 100.7894366958197878, -1.747896926826553843 ) ) ;
#5942=ORIENTED_EDGE ( 'NONE', *, *, #5265, .F. ) ;
#5945=AXIS2_PLACEMENT_3D ( 'NONE', #6016, #4958, #758 ) ;
#5948=ADVANCED_FACE ( 'NONE', ( #3261 ), #7536, .T. ) ;
#5954=AXIS2_PLACEMENT_3D ( 'NONE', #2560, #11946, #3521 ) ;
#5957=CIRCLE ( 'NONE', #5053, 2.000000000000003109 ) ;
#5959=ORIENTED_EDGE ( 'NONE', *, *, #10645, .T. ) ;
#6006=DIRECTION ( 'NONE',  ( 1.000000000000000000, 0.000000000000000000, 0.000000000000000000 ) ) ;
#6008=LINE ( 'NONE', #4947, #11224 ) ;
#6009=FACE_OUTER_BOUND ( 'NONE', #11133, .T. ) ;
#6014=EDGE_LOOP ( 'NONE', ( #5879, #8991, #5314 ) ) ;
#6016=CARTESIAN_POINT ( 'NONE',  ( 39.06230589874905235, 109.5835921350012683, 7.500000000000000000 ) ) ;
#6019=EDGE_CURVE ( 'NONE', #9459, #4575, #1367, .T. ) ;
#6022=DIRECTION ( 'NONE',  ( 0.000000000000000000, -1.000000000000000000, 0.000000000000000000 ) ) ;
#6040=ORIENTED_EDGE ( 'NONE', *, *, #4821, .F. ) ;
#6047=ORIENTED_EDGE ( 'NONE', *, *, #874, .T. ) ;
#6054=DIRECTION ( 'NONE',  ( 1.000000000000000000, -3.851859888774468203E-30, 1.387778780781445676E-15 ) ) ;
#6060=ORIENTED_EDGE ( 'NONE', *, *, #9198, .F. ) ;
#6064=CIRCLE ( 'NONE', #2014, 5.000000000000005329 ) ;
#6075=VERTEX_POINT ( 'NONE', #1239 ) ;
#6076=VECTOR ( 'NONE', #5812, 1000.000000000000000 ) ;
#6081=DIRECTION ( 'NONE',  ( 1.000000000000000000, 0.000000000000000000, 0.000000000000000000 ) ) ;
#6086=AXIS2_PLACEMENT_3D ( 'NONE', #6900, #5867, #2707 ) ;
#6088=VECTOR ( 'NONE', #6218, 999.9999999999998863 ) ;
#6101=( NAMED_UNIT ( * ) SI_UNIT ( $, .STERADIAN. ) SOLID_ANGLE_UNIT ( ) );
#6107=SPHERICAL_SURFACE ( 'NONE', #1471, 5.000000000000000000 ) ;
#6110=ORIENTED_EDGE ( 'NONE', *, *, #5070, .F. ) ;
#6113=ORIENTED_EDGE ( 'NONE', *, *, #7100, .T. ) ;
#6115=ORIENTED_EDGE ( 'NONE', *, *, #13626, .T. ) ;
#6120=ADVANCED_FACE ( 'NONE', ( #6771 ), #13259, .T. ) ;
#6124=CIRCLE ( 'NONE', #13547, 17.49999999999999645 ) ;
#6126=CIRCLE ( 'NONE', #9916, 22.99999999999999645 ) ;
#6135=CARTESIAN_POINT ( 'NONE',  ( 40.81228451836345528, 100.6358150620708329, 0.5000000000000000000 ) ) ;
#6138=DIRECTION ( 'NONE',  ( 0.6000000000000001998, -0.7999999999999999334, 0.000000000000000000 ) ) ;
#6143=DIRECTION ( 'NONE',  ( 0.000000000000000000, 0.000000000000000000, 1.000000000000000000 ) ) ;
#6153=ORIENTED_EDGE ( 'NONE', *, *, #448, .F. ) ;
#6154=VECTOR ( 'NONE', #2350, 1000.000000000000000 ) ;
#6159=DIRECTION ( 'NONE',  ( 1.000000000000000000, 0.000000000000000000, -0.000000000000000000 ) ) ;
#6160=CARTESIAN_POINT ( 'NONE',  ( -42.16244658108818300, 105.4500712252157797, 2.499999999999999556 ) ) ;
#6163=CARTESIAN_POINT ( 'NONE',  ( 42.16244658108818300, 105.4500712252157655, 2.499999999999999556 ) ) ;
#6165=ORIENTED_EDGE ( 'NONE', *, *, #2363, .T. ) ;
#6170=AXIS2_PLACEMENT_3D ( 'NONE', #6466, #94, #2460 ) ;
#6191=DIRECTION ( 'NONE',  ( -0.6000000000000001998, -0.7999999999999999334, 0.000000000000000000 ) ) ;
#6193=DIRECTION ( 'NONE',  ( 0.000000000000000000, 0.000000000000000000, 1.000000000000000000 ) ) ;
#6199=VECTOR ( 'NONE', #9099, 999.9999999999998863 ) ;
#6218=DIRECTION ( 'NONE',  ( -0.6000000000000001998, 0.7999999999999998224, 0.000000000000000000 ) ) ;
#6219=DIRECTION ( 'NONE',  ( 1.000000000000000000, 1.850371707708595549E-15, 0.000000000000000000 ) ) ;
#6224=CARTESIAN_POINT ( 'NONE',  ( -35.06230589874905235, 106.5835921350012825, 2.499999999999999556 ) ) ;
#6227=DIRECTION ( 'NONE',  ( 0.000000000000000000, 0.000000000000000000, 1.000000000000000000 ) ) ;
#6231=ORIENTED_EDGE ( 'NONE', *, *, #9104, .T. ) ;
#6245=AXIS2_PLACEMENT_3D ( 'NONE', #414, #2568, #6907 ) ;
#6257=ORIENTED_EDGE ( 'NONE', *, *, #7321, .T. ) ;
#6262=ADVANCED_FACE ( 'NONE', ( #7712 ), #7914, .F. ) ;
#6273=CARTESIAN_POINT ( 'NONE',  ( 25.00000000000000355, 120.0000000000000142, 7.500000000000000000 ) ) ;
#6276=DIRECTION ( 'NONE',  ( 0.000000000000000000, 1.000000000000000000, 1.734723475976805615E-16 ) ) ;
#6281=CIRCLE ( 'NONE', #8728, 67.49999999999997158 ) ;
#6285=DIRECTION ( 'NONE',  ( 1.000000000000000000, 0.000000000000000000, 0.000000000000000000 ) ) ;
#6291=CIRCLE ( 'NONE', #6954, 12.49999999999999289 ) ;
#6305=DIRECTION ( 'NONE',  ( 1.000000000000000000, 0.000000000000000000, 0.000000000000000000 ) ) ;
#6306=DIRECTION ( 'NONE',  ( -1.000000000000000000, 0.000000000000000000, 0.000000000000000000 ) ) ;
#6314=VERTEX_POINT ( 'NONE', #11366 ) ;
#6315=CARTESIAN_POINT ( 'NONE',  ( 41.49999999999999289, 98.00000000000001421, 7.500000000000000000 ) ) ;
#6318=CARTESIAN_POINT ( 'NONE',  ( -34.79486456029760433, 106.9754367860671778, -2.376147960742915455 ) ) ;
#6324=ORIENTED_EDGE ( 'NONE', *, *, #1794, .T. ) ;
#6326=CARTESIAN_POINT ( 'NONE',  ( 48.00000000000000000, 120.0000000000000142, 2.500000000000000000 ) ) ;
#6330=CARTESIAN_POINT ( 'NONE',  ( -35.04450421339218025, 112.5597086678580609, 2.499999999999999556 ) ) ;
#6338=DIRECTION ( 'NONE',  ( 1.000000000000000000, 0.000000000000000000, 0.000000000000000000 ) ) ;
#6341=EDGE_CURVE ( 'NONE', #2641, #3641, #551, .T. ) ;
#6343=DIRECTION ( 'NONE',  ( 0.000000000000000000, 0.000000000000000000, -1.000000000000000000 ) ) ;
#6344=DIRECTION ( 'NONE',  ( -0.000000000000000000, -0.000000000000000000, -1.000000000000000000 ) ) ;
#6357=CARTESIAN_POINT ( 'NONE',  ( -34.25812584745457201, 108.1980041606221192, 0.000000000000000000 ) ) ;
#6358=ADVANCED_FACE ( 'NONE', ( #9265 ), #787, .T. ) ;
#6364=ORIENTED_EDGE ( 'NONE', *, *, #6885, .F. ) ;
#6387=DIRECTION ( 'NONE',  ( 0.000000000000000000, 0.000000000000000000, 1.000000000000000000 ) ) ;
#6390=ORIENTED_EDGE ( 'NONE', *, *, #8223, .T. ) ;
#6396=CARTESIAN_POINT ( 'NONE',  ( -25.00000000000000355, 120.0000000000000142, 2.500000000000000000 ) ) ;
#6401=CARTESIAN_POINT ( 'NONE',  ( -39.99999999999999289, 120.0000000000000142, 2.500000000000000000 ) ) ;
#6403=CARTESIAN_POINT ( 'NONE',  ( -42.16244658108818300, 105.4500712252157797, -2.500000000000000444 ) ) ;
#6405=TOROIDAL_SURFACE ( 'NONE', #10439, 77.99999999999997158, 2.000000000000000000 ) ;
#6410=AXIS2_PLACEMENT_3D ( 'NONE', #6801, #4692, #4773 ) ;
#6419=DIRECTION ( 'NONE',  ( -0.000000000000000000, -0.000000000000000000, -1.000000000000000000 ) ) ;
#6424=CYLINDRICAL_SURFACE ( 'NONE', #12707, 4.999999999999998224 ) ;
#6426=DIRECTION ( 'NONE',  ( 1.000000000000000000, 0.000000000000000000, -0.000000000000000000 ) ) ;
#6428=ORIENTED_EDGE ( 'NONE', *, *, #5868, .T. ) ;
#6429=EDGE_CURVE ( 'NONE', #9684, #6890, #759, .T. ) ;
#6434=CARTESIAN_POINT ( 'NONE',  ( 42.16244658108818300, 105.4500712252157655, 2.499999999999999556 ) ) ;
#6435=DIRECTION ( 'NONE',  ( 1.000000000000000000, 0.000000000000000000, 0.000000000000000000 ) ) ;
#6443=ORIENTED_EDGE ( 'NONE', *, *, #718, .F. ) ;
#6466=CARTESIAN_POINT ( 'NONE',  ( 25.00000000000000355, 120.0000000000000142, -7.500000000000000000 ) ) ;
#6474=DIRECTION ( 'NONE',  ( -0.000000000000000000, -0.000000000000000000, -1.000000000000000000 ) ) ;
#6479=VERTEX_POINT ( 'NONE', #9477 ) ;
#6480=EDGE_LOOP ( 'NONE', ( #6040, #13390, #7125, #3914, #5058, #13238 ) ) ;
#6482=AXIS2_PLACEMENT_3D ( 'NONE', #8227, #3099, #7368 ) ;
#6486=CYLINDRICAL_SURFACE ( 'NONE', #12886, 14.99999999999999112 ) ;
#6490=DIRECTION ( 'NONE',  ( 0.8907235428302465730, 0.4545454545454549189, -0.000000000000000000 ) ) ;
#6492=CARTESIAN_POINT ( 'NONE',  ( 39.31542348013558552, 101.3376241895501977, 2.435478634890659855 ) ) ;
#6493=DIRECTION ( 'NONE',  ( -0.000000000000000000, -0.000000000000000000, -1.000000000000000000 ) ) ;
#6507=CYLINDRICAL_SURFACE ( 'NONE', #8127, 14.99999999999998934 ) ;
#6509=ORIENTED_EDGE ( 'NONE', *, *, #5651, .T. ) ;
#6511=TOROIDAL_SURFACE ( 'NONE', #7619, 22.99999999999999289, 2.000000000000000000 ) ;
#6517=ORIENTED_EDGE ( 'NONE', *, *, #2737, .T. ) ;
#6519=DIRECTION ( 'NONE',  ( 0.000000000000000000, 0.000000000000000000, 1.000000000000000000 ) ) ;
#6522=AXIS2_PLACEMENT_3D ( 'NONE', #12836, #8868, #9588 ) ;
#6523=CARTESIAN_POINT ( 'NONE',  ( 39.64464840659818634, 101.1283747906780803, -2.297097423097429925 ) ) ;
#6558=CARTESIAN_POINT ( 'NONE',  ( 34.58386302044579708, 107.3580618547655803, -2.150514425741560931 ) ) ;
#6559=DIRECTION ( 'NONE',  ( 0.000000000000000000, 0.000000000000000000, 1.000000000000000000 ) ) ;
#6564=DIRECTION ( 'NONE',  ( 1.000000000000000000, -1.850371707708595154E-15, 0.000000000000000000 ) ) ;
#6570=UNCERTAINTY_MEASURE_WITH_UNIT (LENGTH_MEASURE( 1.000000000000000082E-05 ), #12413, 'distance_accuracy_value', 'NONE');
#6572=CIRCLE ( 'NONE', #12647, 22.49999999999999289 ) ;
#6580=FACE_OUTER_BOUND ( 'NONE', #8942, .T. ) ;
#6586=ORIENTED_EDGE ( 'NONE', *, *, #13626, .F. ) ;
#6587=AXIS2_PLACEMENT_3D ( 'NONE', #12837, #11761, #4321 ) ;
#6590=AXIS2_PLACEMENT_3D ( 'NONE', #5093, #3905, #11201 ) ;
#6592=CARTESIAN_POINT ( 'NONE',  ( -39.06230589874905235, 109.5835921350012683, -2.499999999999999556 ) ) ;
#6597=ADVANCED_FACE ( 'NONE', ( #1624 ), #8995, .T. ) ;
#6598=DIRECTION ( 'NONE',  ( 1.000000000000000000, 0.000000000000000000, 0.000000000000000000 ) ) ;
#6606=ADVANCED_FACE ( 'NONE', ( #10116 ), #4111, .T. ) ;
#6608=ADVANCED_FACE ( 'NONE', ( #11089 ), #8921, .F. ) ;
#6612=EDGE_LOOP ( 'NONE', ( #2308, #177, #3745, #1422 ) ) ;
#6622=CARTESIAN_POINT ( 'NONE',  ( 34.91511737228310608, 106.7798435036222884, -2.458454180825599078 ) ) ;
#6625=DIRECTION ( 'NONE',  ( 1.000000000000000000, -8.163404592832038896E-16, 0.000000000000000000 ) ) ;
#6633=DIRECTION ( 'NONE',  ( -0.000000000000000000, -0.000000000000000000, -1.000000000000000000 ) ) ;
#6636=PRODUCT_CONTEXT ( 'NONE', #5047, 'mechanical' ) ;
#6638=CARTESIAN_POINT ( 'NONE',  ( -31.81818181818181657, 133.3608531424536920, 2.500000000000000000 ) ) ;
#6641=AXIS2_PLACEMENT_3D ( 'NONE', #6160, #832, #2076 ) ;
#6642=DIRECTION ( 'NONE',  ( -0.000000000000000000, -0.000000000000000000, -1.000000000000000000 ) ) ;
#6646=AXIS2_PLACEMENT_3D ( 'NONE', #10000, #410, #4663 ) ;
#6672=ORIENTED_EDGE ( 'NONE', *, *, #1809, .F. ) ;
#6680=DIRECTION ( 'NONE',  ( -0.000000000000000000, -0.000000000000000000, -1.000000000000000000 ) ) ;
#6690=CARTESIAN_POINT ( 'NONE',  ( 35.06230589874905235, 106.5835921350012967, -2.486789939184903986 ) ) ;
#6692=CARTESIAN_POINT ( 'NONE',  ( -39.42607625790187598, 101.2633694847512800, -2.396914520158672790 ) ) ;
#6693=CARTESIAN_POINT ( 'NONE',  ( 40.79557129359545797, 100.6404192164768716, 0.7730400384045159612 ) ) ;
#6698=VERTEX_POINT ( 'NONE', #840 ) ;
#6702=ORIENTED_EDGE ( 'NONE', *, *, #12808, .F. ) ;
#6706=DIRECTION ( 'NONE',  ( 0.4545454545454548634, 0.8907235428302464619, 0.000000000000000000 ) ) ;
#6716=VERTEX_POINT ( 'NONE', #13708 ) ;
#6717=AXIS2_PLACEMENT_3D ( 'NONE', #13727, #6193, #4992 ) ;
#6718=LINE ( 'NONE', #5590, #6076 ) ;
#6719=EDGE_CURVE ( 'NONE', #13844, #973, #5239, .T. ) ;
#6726=CARTESIAN_POINT ( 'NONE',  ( 48.00000000000000000, 120.0000000000000142, -2.500000000000000000 ) ) ;
#6727=CIRCLE ( 'NONE', #29, 2.000000000000003997 ) ;
#6745=DIRECTION ( 'NONE',  ( 1.000000000000000000, 0.000000000000000000, 0.000000000000000000 ) ) ;
#6752=VERTEX_POINT ( 'NONE', #2215 ) ;
#6759=LINE ( 'NONE', #12088, #13117 ) ;
#6763=CARTESIAN_POINT ( 'NONE',  ( 34.37544226909922429, 107.8407100838017385, -1.642507177281958830 ) ) ;
#6766=DIRECTION ( 'NONE',  ( 1.000000000000000000, 0.000000000000000000, 0.000000000000000000 ) ) ;
#6771=FACE_OUTER_BOUND ( 'NONE', #3814, .T. ) ;
#6776=VERTEX_POINT ( 'NONE', #2017 ) ;
#6780=DIRECTION ( 'NONE',  ( 0.000000000000000000, 0.000000000000000000, 1.000000000000000000 ) ) ;
#6781=EDGE_CURVE ( 'NONE', #4883, #369, #5031, .T. ) ;
#6787=EDGE_CURVE ( 'NONE', #624, #3971, #9288, .T. ) ;
#6796=PRESENTATION_STYLE_ASSIGNMENT (( #2519 ) ) ;
#6798=EDGE_CURVE ( 'NONE', #9003, #10135, #9798, .T. ) ;
#6801=CARTESIAN_POINT ( 'NONE',  ( 25.00000000000000355, 120.0000000000000142, 2.499999999999999556 ) ) ;
#6807=ORIENTED_EDGE ( 'NONE', *, *, #10710, .T. ) ;
#6823=ORIENTED_EDGE ( 'NONE', *, *, #8070, .T. ) ;
#6838=DIRECTION ( 'NONE',  ( 1.000000000000000000, 0.000000000000000000, 0.000000000000000000 ) ) ;
#6843=CYLINDRICAL_SURFACE ( 'NONE', #12863, 12.49999999999999112 ) ;
#6848=CIRCLE ( 'NONE', #2591, 12.49999999999998757 ) ;
#6857=DIRECTION ( 'NONE',  ( -0.000000000000000000, -0.000000000000000000, -1.000000000000000000 ) ) ;
#6859=CIRCLE ( 'NONE', #11115, 5.000000000000001776 ) ;
#6863=ORIENTED_EDGE ( 'NONE', *, *, #6341, .T. ) ;
#6864=EDGE_LOOP ( 'NONE', ( #13367, #3721, #3493, #9085 ) ) ;
#6865=EDGE_CURVE ( 'NONE', #7675, #780, #574, .T. ) ;
#6868=ORIENTED_EDGE ( 'NONE', *, *, #1809, .T. ) ;
#6876=CARTESIAN_POINT ( 'NONE',  ( -34.33120614476065668, 107.9646345552176001, 1.436946644489085267 ) ) ;
#6878=VERTEX_POINT ( 'NONE', #138 ) ;
#6881=CARTESIAN_POINT ( 'NONE',  ( 0.000000000000000000, 71.01020514433645303, -2.499999999999998668 ) ) ;
#6883=ORIENTED_EDGE ( 'NONE', *, *, #2653, .F. ) ;
#6885=EDGE_CURVE ( 'NONE', #9880, #8180, #11054, .T. ) ;
#6890=VERTEX_POINT ( 'NONE', #13112 ) ;
#6894=CARTESIAN_POINT ( 'NONE',  ( 38.16244658108818300, 102.4500712252157655, 2.500000000000000000 ) ) ;
#6900=CARTESIAN_POINT ( 'NONE',  ( -35.22727272727274794, 140.0412797136805523, 2.499999999999999556 ) ) ;
#6904=FACE_OUTER_BOUND ( 'NONE', #2272, .T. ) ;
#6907=DIRECTION ( 'NONE',  ( 1.000000000000000000, 0.000000000000000000, -1.387778780781446464E-15 ) ) ;
#6910=ORIENTED_EDGE ( 'NONE', *, *, #10380, .T. ) ;
#6923=ORIENTED_EDGE ( 'NONE', *, *, #11244, .F. ) ;
#6930=FACE_OUTER_BOUND ( 'NONE', #599, .T. ) ;
#6938=CIRCLE ( 'NONE', #9188, 12.49999999999998757 ) ;
#6946=ORIENTED_EDGE ( 'NONE', *, *, #5232, .T. ) ;
#6954=AXIS2_PLACEMENT_3D ( 'NONE', #3390, #2488, #3323 ) ;
#6961=ORIENTED_EDGE ( 'NONE', *, *, #10786, .F. ) ;
#6966=EDGE_CURVE ( 'NONE', #3876, #4722, #3000, .T. ) ;
#6975=DIRECTION ( 'NONE',  ( 1.000000000000000000, 0.000000000000000000, 0.000000000000000000 ) ) ;
#6980=CARTESIAN_POINT ( 'NONE',  ( -38.89115197531749857, 101.6687180808697377, 2.500000000000000000 ) ) ;
#6986=CARTESIAN_POINT ( 'NONE',  ( 10.99999999999999289, 147.0000000000000284, -2.499999999999999556 ) ) ;
#6994=DIRECTION ( 'NONE',  ( 1.000000000000000000, 0.000000000000000000, 0.000000000000000000 ) ) ;
#6997=CARTESIAN_POINT ( 'NONE',  ( -32.72727272727271952, 135.1423002281141805, -0.5000000000000000000 ) ) ;
#6998=DIRECTION ( 'NONE',  ( 1.000000000000000000, 0.000000000000000000, 0.000000000000000000 ) ) ;
#7005=CARTESIAN_POINT ( 'NONE',  ( -32.72727272727271952, 135.1423002281141805, 2.500000000000000000 ) ) ;
#7015=ORIENTED_EDGE ( 'NONE', *, *, #4063, .F. ) ;
#7028=VERTEX_POINT ( 'NONE', #1735 ) ;
#7039=CARTESIAN_POINT ( 'NONE',  ( 25.00000000000000355, 120.0000000000000142, -2.499999999999998668 ) ) ;
#7048=DIRECTION ( 'NONE',  ( 0.000000000000000000, 0.000000000000000000, 1.000000000000000000 ) ) ;
#7059=EDGE_CURVE ( 'NONE', #5379, #10090, #7095, .T. ) ;
#7060=DIRECTION ( 'NONE',  ( 1.000000000000000000, 0.000000000000000000, 0.000000000000000000 ) ) ;
#7061=CARTESIAN_POINT ( 'NONE',  ( -38.89115197531749857, 101.6687180808697377, 2.500000000000000000 ) ) ;
#7070=ORIENTED_EDGE ( 'NONE', *, *, #4063, .T. ) ;
#7078=CARTESIAN_POINT ( 'NONE',  ( -35.22727272727274794, 140.0412797136805523, -7.500000000000000000 ) ) ;
#7082=EDGE_LOOP ( 'NONE', ( #12835, #2172, #9476, #5136 ) ) ;
#7084=ORIENTED_EDGE ( 'NONE', *, *, #2119, .F. ) ;
#7086=CARTESIAN_POINT ( 'NONE',  ( 25.00000000000000355, 120.0000000000000142, -2.500000000000000000 ) ) ;
#7095=B_SPLINE_CURVE_WITH_KNOTS ( 'NONE', 3,
 ( #3321, #8655, #2487, #2409, #8718, #11035, #3387, #6763, #11881, #8870, #1435, #6558, #13025, #10753, #6622, #6690 ),
 .UNSPECIFIED., .F., .F.,
 ( 4, 2, 2, 2, 2, 2, 2, 4 ),
 ( 1.969947839904427242E-07, 0.0003650593540107671415, 0.0007299217132375439157, 0.001094784072464320690, 0.001459646431691097356, 0.001824508790917874239, 0.002189371150144650904, 0.002919095868598195129 ),
 .UNSPECIFIED. ) ;
#7100=EDGE_CURVE ( 'NONE', #5579, #9616, #11204, .T. ) ;
#7106=CARTESIAN_POINT ( 'NONE',  ( -32.72727272727271952, 135.1423002281141805, -2.500000000000000000 ) ) ;
#7118=DIRECTION ( 'NONE',  ( 1.000000000000000000, 0.000000000000000000, 0.000000000000000000 ) ) ;
#7123=EDGE_CURVE ( 'NONE', #6716, #3641, #8345, .T. ) ;
#7125=ORIENTED_EDGE ( 'NONE', *, *, #1794, .F. ) ;
#7136=CIRCLE ( 'NONE', #10487, 2.000000000000000000 ) ;
#7144=CARTESIAN_POINT ( 'NONE',  ( 34.33153323985096250, 107.9636705364999472, 1.438784920770795894 ) ) ;
#7153=CIRCLE ( 'NONE', #6482, 4.999999999999998224 ) ;
#7167=VERTEX_POINT ( 'NONE', #3890 ) ;
#7175=TOROIDAL_SURFACE ( 'NONE', #10978, 22.49999999999998934, 5.000000000000000000 ) ;
#7180=CARTESIAN_POINT ( 'NONE',  ( 0.000000000000000000, 71.01020514433645303, 0.5000000000000000000 ) ) ;
#7186=CIRCLE ( 'NONE', #1598, 12.49999999999999289 ) ;
#7195=ADVANCED_FACE ( 'NONE', ( #4812 ), #11190, .F. ) ;
#7210=CARTESIAN_POINT ( 'NONE',  ( 34.25812584745457201, 108.1980041606221050, 0.5000000000000000000 ) ) ;
#7222=EDGE_CURVE ( 'NONE', #13399, #1557, #11417, .T. ) ;
#7229=FACE_OUTER_BOUND ( 'NONE', #1731, .T. ) ;
#7235=VERTEX_POINT ( 'NONE', #12315 ) ;
#7251=DIRECTION ( 'NONE',  ( 0.8907235428302444635, 0.4545454545454587492, 0.000000000000000000 ) ) ;
#7257=ORIENTED_EDGE ( 'NONE', *, *, #13518, .T. ) ;
#7266=DIRECTION ( 'NONE',  ( -0.000000000000000000, -0.000000000000000000, -1.000000000000000000 ) ) ;
#7277=CARTESIAN_POINT ( 'NONE',  ( 34.27523635402735636, 108.1397967565350200, 0.9870360185550118848 ) ) ;
#7288=EDGE_CURVE ( 'NONE', #7028, #6075, #7826, .T. ) ;
#7302=DIRECTION ( 'NONE',  ( 0.8000000000000008216, 0.5999999999999988676, -4.163336342344329138E-15 ) ) ;
#7307=ORIENTED_EDGE ( 'NONE', *, *, #1730, .T. ) ;
#7311=FACE_OUTER_BOUND ( 'NONE', #8319, .T. ) ;
#7314=CARTESIAN_POINT ( 'NONE',  ( -36.36363636363635976, 142.2680885707561629, 2.500000000000000000 ) ) ;
#7318=CARTESIAN_POINT ( 'NONE',  ( 52.49999999999999289, 120.0000000000000142, 2.499999999999999556 ) ) ;
#7321=EDGE_CURVE ( 'NONE', #8040, #13223, #8287, .T. ) ;
#7337=CARTESIAN_POINT ( 'NONE',  ( 34.79486456029760433, 106.9754367860671778, 2.376147960742919452 ) ) ;
#7343=EDGE_LOOP ( 'NONE', ( #1843, #8897, #12421, #12011 ) ) ;
#7347=ORIENTED_EDGE ( 'NONE', *, *, #11809, .T. ) ;
#7353=CARTESIAN_POINT ( 'NONE',  ( -36.50000000000000000, 113.0000000000000142, 2.499999999999999556 ) ) ;
#7360=EDGE_CURVE ( 'NONE', #9139, #2097, #3044, .T. ) ;
#7364=ORIENTED_EDGE ( 'NONE', *, *, #1364, .F. ) ;
#7365=ORIENTED_EDGE ( 'NONE', *, *, #9772, .F. ) ;
#7368=DIRECTION ( 'NONE',  ( -0.4545454545454548634, 0.8907235428302464619, 0.000000000000000000 ) ) ;
#7382=EDGE_CURVE ( 'NONE', #2641, #780, #8711, .T. ) ;
#7384=CARTESIAN_POINT ( 'NONE',  ( -35.45454545454546036, 140.4866414850956744, -0.5000000000000000000 ) ) ;
#7385=CARTESIAN_POINT ( 'NONE',  ( 30.68181818181819054, 131.1340442853780530, 2.499999999999999556 ) ) ;
#7389=ORIENTED_EDGE ( 'NONE', *, *, #2653, .T. ) ;
#7390=TOROIDAL_SURFACE ( 'NONE', #5365, 17.49999999999999645, 5.000000000000000000 ) ;
#7399=CARTESIAN_POINT ( 'NONE',  ( -10.00000000000000711, 140.0000000000000000, 2.500000000000000000 ) ) ;
#7408=CIRCLE ( 'NONE', #3159, 5.000000000000004441 ) ;
#7412=ORIENTED_EDGE ( 'NONE', *, *, #5750, .F. ) ;
#7421=AXIS2_PLACEMENT_3D ( 'NONE', #10734, #12726, #2115 ) ;
#7422=VERTEX_POINT ( 'NONE', #11596 ) ;
#7423=CARTESIAN_POINT ( 'NONE',  ( 35.06230589874905235, 106.5835921350012967, -2.486789939184903986 ) ) ;
#7424=CARTESIAN_POINT ( 'NONE',  ( -25.00000000000000355, 120.0000000000000142, 2.499999999999999556 ) ) ;
#7431=DIRECTION ( 'NONE',  ( 0.4545454545454531425, 0.8907235428302472391, 0.000000000000000000 ) ) ;
#7436=ORIENTED_EDGE ( 'NONE', *, *, #11056, .F. ) ;
#7443=CIRCLE ( 'NONE', #1858, 2.000000000000000000 ) ;
#7467=AXIS2_PLACEMENT_3D ( 'NONE', #8214, #855, #5119 ) ;
#7474=DIRECTION ( 'NONE',  ( 1.000000000000000000, 0.000000000000000000, 0.000000000000000000 ) ) ;
#7486=AXIS2_PLACEMENT_3D ( 'NONE', #5158, #12887, #12819 ) ;
#7488=ORIENTED_EDGE ( 'NONE', *, *, #13161, .F. ) ;
#7490=AXIS2_PLACEMENT_3D ( 'NONE', #10483, #12607, #4230 ) ;
#7495=DIRECTION ( 'NONE',  ( 0.000000000000000000, 0.000000000000000000, 1.000000000000000000 ) ) ;
#7496=CARTESIAN_POINT ( 'NONE',  ( 0.000000000000000000, 71.01020514433645303, -2.499999999999998668 ) ) ;
#7515=AXIS2_PLACEMENT_3D ( 'NONE', #11474, #1866, #8118 ) ;
#7519=DIRECTION ( 'NONE',  ( -0.5999999999999989786, -0.8000000000000008216, 0.000000000000000000 ) ) ;
#7525=VERTEX_POINT ( 'NONE', #11796 ) ;
#7526=DIRECTION ( 'NONE',  ( -0.000000000000000000, -0.000000000000000000, -1.000000000000000000 ) ) ;
#7531=EDGE_CURVE ( 'NONE', #11542, #397, #10313, .T. ) ;
#7532=CARTESIAN_POINT ( 'NONE',  ( -45.97632359910779343, 102.2167537197081799, 2.499999999999999556 ) ) ;
#7536=PLANE ( 'NONE',  #298 ) ;
#7549=ADVANCED_FACE ( 'NONE', ( #7229 ), #2925, .T. ) ;
#7550=ORIENTED_EDGE ( 'NONE', *, *, #6781, .T. ) ;
#7592=ORIENTED_EDGE ( 'NONE', *, *, #4980, .F. ) ;
#7600=DIRECTION ( 'NONE',  ( -0.000000000000000000, -0.000000000000000000, -1.000000000000000000 ) ) ;
#7601=CARTESIAN_POINT ( 'NONE',  ( 40.05714107113524847, 100.9137399031062898, 2.016203456813714379 ) ) ;
#7606=CARTESIAN_POINT ( 'NONE',  ( -37.50000000000000000, 120.0000000000000142, 2.499999999999999556 ) ) ;
#7608=ORIENTED_EDGE ( 'NONE', *, *, #4821, .T. ) ;
#7612=ORIENTED_EDGE ( 'NONE', *, *, #12336, .T. ) ;
#7614=AXIS2_PLACEMENT_3D ( 'NONE', #7670, #3525, #11036 ) ;
#7619=AXIS2_PLACEMENT_3D ( 'NONE', #12694, #1747, #6305 ) ;
#7624=EDGE_CURVE ( 'NONE', #6698, #12375, #13491, .T. ) ;
#7634=VECTOR ( 'NONE', #8168, 1000.000000000000000 ) ;
#7635=CARTESIAN_POINT ( 'NONE',  ( -34.37593967123855521, 107.8393652239837337, -1.644494279733349718 ) ) ;
#7638=DIRECTION ( 'NONE',  ( 0.8000000000000024869, 0.5999999999999966471, 0.000000000000000000 ) ) ;
#7641=ORIENTED_EDGE ( 'NONE', *, *, #12004, .F. ) ;
#7647=CARTESIAN_POINT ( 'NONE',  ( 0.000000000000000000, 71.01020514433645303, 0.5000000000000000000 ) ) ;
#7664=CIRCLE ( 'NONE', #12163, 12.49999999999998757 ) ;
#7669=DIRECTION ( 'NONE',  ( 1.000000000000000000, 0.000000000000000000, 0.000000000000000000 ) ) ;
#7670=CARTESIAN_POINT ( 'NONE',  ( -29.00000000000000000, 123.0000000000000142, -2.499999999999999556 ) ) ;
#7675=VERTEX_POINT ( 'NONE', #11842 ) ;
#7698=CARTESIAN_POINT ( 'NONE',  ( -25.00000000000000355, 120.0000000000000142, 2.499999999999999556 ) ) ;
#7702=CARTESIAN_POINT ( 'NONE',  ( 39.06230589874905235, 109.5835921350012825, -7.500000000000000000 ) ) ;
#7704=VECTOR ( 'NONE', #5656, 999.9999999999998863 ) ;
#7708=TOROIDAL_SURFACE ( 'NONE', #5254, 22.49999999999998934, 5.000000000000000000 ) ;
#7712=FACE_OUTER_BOUND ( 'NONE', #846, .T. ) ;
#7725=ORIENTED_EDGE ( 'NONE', *, *, #12353, .F. ) ;
#7726=AXIS2_PLACEMENT_3D ( 'NONE', #10185, #453, #4859 ) ;
#7728=AXIS2_PLACEMENT_3D ( 'NONE', #12064, #12864, #2176 ) ;
#7733=CIRCLE ( 'NONE', #4381, 24.99999999999998934 ) ;
#7739=DIRECTION ( 'NONE',  ( 1.000000000000000000, 0.000000000000000000, 0.000000000000000000 ) ) ;
#7756=ORIENTED_EDGE ( 'NONE', *, *, #2310, .F. ) ;
#7760=ORIENTED_EDGE ( 'NONE', *, *, #9201, .T. ) ;
#7770=ORIENTED_EDGE ( 'NONE', *, *, #3425, .T. ) ;
#7773=EDGE_CURVE ( 'NONE', #9005, #397, #6938, .T. ) ;
#7787=CARTESIAN_POINT ( 'NONE',  ( 36.36363636363638108, 142.2680885707561629, -0.5000000000000000000 ) ) ;
#7798=ORIENTED_EDGE ( 'NONE', *, *, #12372, .F. ) ;
#7799=ORIENTED_EDGE ( 'NONE', *, *, #2071, .F. ) ;
#7800=DIRECTION ( 'NONE',  ( -0.6000000000000001998, 0.7999999999999998224, 0.000000000000000000 ) ) ;
#7805=EDGE_CURVE ( 'NONE', #1833, #9552, #6064, .T. ) ;
#7809=CARTESIAN_POINT ( 'NONE',  ( 0.000000000000000000, 71.01020514433645303, -2.500000000000000000 ) ) ;
#7810=FACE_OUTER_BOUND ( 'NONE', #6480, .T. ) ;
#7819=AXIS2_PLACEMENT_3D ( 'NONE', #4029, #8316, #6219 ) ;
#7826=CIRCLE ( 'NONE', #11859, 17.49999999999999645 ) ;
#7831=VECTOR ( 'NONE', #6680, 1000.000000000000000 ) ;
#7835=FACE_OUTER_BOUND ( 'NONE', #1688, .T. ) ;
#7856=CARTESIAN_POINT ( 'NONE',  ( 35.22727272727274084, 140.0412797136805523, -7.500000000000000000 ) ) ;
#7862=CIRCLE ( 'NONE', #6086, 4.999999999999998224 ) ;
#7869=CARTESIAN_POINT ( 'NONE',  ( 42.16244658108817589, 105.4500712252157655, -2.499999999999999556 ) ) ;
#7871=ORIENTED_EDGE ( 'NONE', *, *, #11677, .F. ) ;
#7877=TOROIDAL_SURFACE ( 'NONE', #8334, 22.99999999999999289, 2.000000000000000000 ) ;
#7882=VERTEX_POINT ( 'NONE', #9183 ) ;
#7889=CARTESIAN_POINT ( 'NONE',  ( 41.99999999999999289, 120.0000000000000142, 0.5000000000000000000 ) ) ;
#7893=DIRECTION ( 'NONE',  ( 0.000000000000000000, 0.000000000000000000, 1.000000000000000000 ) ) ;
#7914=TOROIDAL_SURFACE ( 'NONE', #12850, 71.99999999999998579, 2.000000000000000000 ) ;
#7915=DIRECTION ( 'NONE',  ( 0.000000000000000000, 0.000000000000000000, 1.000000000000000000 ) ) ;
#7917=ADVANCED_FACE ( 'NONE', ( #8204 ), #6511, .F. ) ;
#7920=ORIENTED_EDGE ( 'NONE', *, *, #13254, .F. ) ;
#7925=DIRECTION ( 'NONE',  ( -0.6466635011015237078, -0.7627754036039179342, -0.000000000000000000 ) ) ;
#7929=EDGE_LOOP ( 'NONE', ( #9542, #797, #12232, #1117 ) ) ;
#7933=AXIS2_PLACEMENT_3D ( 'NONE', #7086, #377, #10111 ) ;
#7935=CARTESIAN_POINT ( 'NONE',  ( 0.000000000000000000, 71.01020514433645303, 2.500000000000000000 ) ) ;
#7946=AXIS2_PLACEMENT_3D ( 'NONE', #11879, #9920, #4659 ) ;
#7952=DIRECTION ( 'NONE',  ( 0.000000000000000000, 0.000000000000000000, 1.000000000000000000 ) ) ;
#7960=CARTESIAN_POINT ( 'NONE',  ( -35.06230589874905235, 106.5835921350012825, 7.500000000000000000 ) ) ;
#7961=VECTOR ( 'NONE', #7800, 999.9999999999998863 ) ;
#7964=CARTESIAN_POINT ( 'NONE',  ( -40.81228451836347659, 100.6358150620708614, -0.6381026355483951917 ) ) ;
#7972=AXIS2_PLACEMENT_3D ( 'NONE', #9623, #13739, #10602 ) ;
#7983=CARTESIAN_POINT ( 'NONE',  ( -40.24692185806993194, 100.8304034607652255, 1.836112450589438838 ) ) ;
#7995=AXIS2_PLACEMENT_3D ( 'NONE', #8671, #12838, #6435 ) ;
#8000=CARTESIAN_POINT ( 'NONE',  ( -39.99999999999999289, 120.0000000000000142, -0.5000000000000000000 ) ) ;
#8015=DIRECTION ( 'NONE',  ( -0.000000000000000000, -0.000000000000000000, -1.000000000000000000 ) ) ;
#8030=DIRECTION ( 'NONE',  ( 0.000000000000000000, -1.000000000000000000, 0.000000000000000000 ) ) ;
#8038=FACE_OUTER_BOUND ( 'NONE', #8581, .T. ) ;
#8040=VERTEX_POINT ( 'NONE', #3824 ) ;
#8043=ORIENTED_EDGE ( 'NONE', *, *, #12876, .F. ) ;
#8044=ORIENTED_EDGE ( 'NONE', *, *, #2592, .F. ) ;
#8045=CARTESIAN_POINT ( 'NONE',  ( -25.00000000000000355, 120.0000000000000142, 2.499999999999999556 ) ) ;
#8048=CARTESIAN_POINT ( 'NONE',  ( -40.49366238756161351, 100.7360090884195500, 1.526167340029800146 ) ) ;
#8063=FACE_OUTER_BOUND ( 'NONE', #6014, .T. ) ;
#8066=EDGE_LOOP ( 'NONE', ( #3211, #9039, #13373, #10597 ) ) ;
#8070=EDGE_CURVE ( 'NONE', #9516, #1833, #11214, .T. ) ;
#8073=CIRCLE ( 'NONE', #12570, 27.49999999999999289 ) ;
#8076=EDGE_CURVE ( 'NONE', #7525, #4575, #6727, .T. ) ;
#8087=CIRCLE ( 'NONE', #10315, 4.999999999999998224 ) ;
#8106=DIRECTION ( 'NONE',  ( 1.000000000000000000, 0.000000000000000000, 0.000000000000000000 ) ) ;
#8115=ADVANCED_FACE ( 'NONE', ( #749 ), #3591, .T. ) ;
#8118=DIRECTION ( 'NONE',  ( 1.000000000000000000, -5.551115123125785069E-15, 0.000000000000000000 ) ) ;
#8124=DIRECTION ( 'NONE',  ( 0.8907235428302453517, -0.4545454545454570838, 0.000000000000000000 ) ) ;
#8125=ORIENTED_EDGE ( 'NONE', *, *, #10710, .F. ) ;
#8127=AXIS2_PLACEMENT_3D ( 'NONE', #10771, #5443, #9731 ) ;
#8144=ORIENTED_EDGE ( 'NONE', *, *, #11056, .T. ) ;
#8147=ADVANCED_FACE ( 'NONE', ( #6904 ), #12578, .T. ) ;
#8154=DIRECTION ( 'NONE',  ( -0.000000000000000000, -0.000000000000000000, -1.000000000000000000 ) ) ;
#8156=ORIENTED_EDGE ( 'NONE', *, *, #3023, .T. ) ;
#8157=ORIENTED_EDGE ( 'NONE', *, *, #12356, .T. ) ;
#8163=DIRECTION ( 'NONE',  ( 0.8035603370713739757, 0.5952233065713573579, 0.000000000000000000 ) ) ;
#8164=FACE_OUTER_BOUND ( 'NONE', #8066, .T. ) ;
#8166=DIRECTION ( 'NONE',  ( 0.000000000000000000, 1.000000000000000000, 2.775557561562888984E-15 ) ) ;
#8168=DIRECTION ( 'NONE',  ( -0.000000000000000000, -0.000000000000000000, 1.000000000000000000 ) ) ;
#8176=EDGE_CURVE ( 'NONE', #10854, #10350, #6008, .T. ) ;
#8177=EDGE_LOOP ( 'NONE', ( #3671, #72, #7798, #2294, #5036 ) ) ;
#8180=VERTEX_POINT ( 'NONE', #13544 ) ;
#8181=TOROIDAL_SURFACE ( 'NONE', #13362, 16.99999999999998934, 2.000000000000000000 ) ;
#8193=AXIS2_PLACEMENT_3D ( 'NONE', #1409, #10931, #382 ) ;
#8199=PRODUCT_DEFINITION_FORMATION_WITH_SPECIFIED_SOURCE ( 'ANY', '', #3279, .NOT_KNOWN. ) ;
#8200=ORIENTED_EDGE ( 'NONE', *, *, #7222, .T. ) ;
#8204=FACE_OUTER_BOUND ( 'NONE', #1528, .T. ) ;
#8210=DIRECTION ( 'NONE',  ( 1.000000000000000000, 0.000000000000000000, 0.000000000000000000 ) ) ;
#8212=CARTESIAN_POINT ( 'NONE',  ( 39.06230589874904524, 109.5835921350012683, -2.499999999999998668 ) ) ;
#8214=CARTESIAN_POINT ( 'NONE',  ( 39.06230589874905235, 109.5835921350012683, -2.499999999999999556 ) ) ;
#8223=EDGE_CURVE ( 'NONE', #6698, #8382, #8735, .T. ) ;
#8225=ADVANCED_FACE ( 'NONE', ( #5346 ), #1013, .T. ) ;
#8227=CARTESIAN_POINT ( 'NONE',  ( -32.95454545454546746, 135.5876619995293311, -2.499999999999998668 ) ) ;
#8231=PLANE ( 'NONE',  #13294 ) ;
#8241=ORIENTED_EDGE ( 'NONE', *, *, #5748, .F. ) ;
#8243=EDGE_CURVE ( 'NONE', #12375, #9005, #9435, .T. ) ;
#8253=CARTESIAN_POINT ( 'NONE',  ( 0.000000000000000000, 71.01020514433645303, 7.500000000000000000 ) ) ;
#8258=EDGE_LOOP ( 'NONE', ( #12814, #8582, #507, #3981, #5833, #1898 ) ) ;
#8266=CARTESIAN_POINT ( 'NONE',  ( -25.00000000000000355, 120.0000000000000142, 7.500000000000000000 ) ) ;
#8287=CIRCLE ( 'NONE', #4696, 5.000000000000000000 ) ;
#8301=CIRCLE ( 'NONE', #3360, 4.999999999999997335 ) ;
#8302=CARTESIAN_POINT ( 'NONE',  ( 41.49999999999999289, 98.00000000000001421, 7.500000000000000000 ) ) ;
#8304=DIRECTION ( 'NONE',  ( 0.000000000000000000, 0.000000000000000000, 1.000000000000000000 ) ) ;
#8309=DIRECTION ( 'NONE',  ( -0.7999999999999996003, -0.6000000000000007550, -8.673617379884038430E-16 ) ) ;
#8316=DIRECTION ( 'NONE',  ( -0.000000000000000000, -0.000000000000000000, -1.000000000000000000 ) ) ;
#8319=EDGE_LOOP ( 'NONE', ( #10838, #8557, #3115, #355, #4837 ) ) ;
#8320=CARTESIAN_POINT ( 'NONE',  ( -32.50000000000000000, 110.0000000000000142, -2.499999999999999556 ) ) ;
#8328=EDGE_CURVE ( 'NONE', #9552, #2984, #13026, .T. ) ;
#8330=DIRECTION ( 'NONE',  ( 0.6000000000000001998, 0.7999999999999998224, -0.000000000000000000 ) ) ;
#8333=ORIENTED_EDGE ( 'NONE', *, *, #12378, .T. ) ;
#8334=AXIS2_PLACEMENT_3D ( 'NONE', #12197, #7915, #13200 ) ;
#8345=CIRCLE ( 'NONE', #11914, 22.99999999999999289 ) ;
#8354=DIRECTION ( 'NONE',  ( 0.8035603370713739757, -0.5952233065713573579, 0.000000000000000000 ) ) ;
#8360=EDGE_CURVE ( 'NONE', #4722, #7675, #1361, .T. ) ;
#8370=DIRECTION ( 'NONE',  ( 0.000000000000000000, 1.000000000000000000, 1.734723475976805615E-16 ) ) ;
#8379=ORIENTED_EDGE ( 'NONE', *, *, #12704, .T. ) ;
#8382=VERTEX_POINT ( 'NONE', #8927 ) ;
#8383=AXIS2_PLACEMENT_3D ( 'NONE', #6881, #11159, #13374 ) ;
#8391=AXIS2_PLACEMENT_3D ( 'NONE', #3539, #6780, #12186 ) ;
#8393=AXIS2_PLACEMENT_3D ( 'NONE', #1167, #5424, #5160 ) ;
#8395=CIRCLE ( 'NONE', #2338, 5.000000000000000000 ) ;
#8411=CARTESIAN_POINT ( 'NONE',  ( -42.16244658108818300, 105.4500712252157655, -2.499999999999999556 ) ) ;
#8413=EDGE_CURVE ( 'NONE', #6698, #8935, #4355, .T. ) ;
#8421=ADVANCED_FACE ( 'NONE', ( #8704 ), #2037, .F. ) ;
#8429=EDGE_LOOP ( 'NONE', ( #7799, #823, #7488, #9740, #4776, #6443 ) ) ;
#8450=VERTEX_POINT ( 'NONE', #7787 ) ;
#8451=DIRECTION ( 'NONE',  ( -0.000000000000000000, -0.000000000000000000, -1.000000000000000000 ) ) ;
#8452=CARTESIAN_POINT ( 'NONE',  ( 25.00000000000000355, 120.0000000000000142, 2.500000000000000000 ) ) ;
#8453=CARTESIAN_POINT ( 'NONE',  ( 41.50000000000000711, 98.00000000000000000, -2.499999999999999556 ) ) ;
#8465=CARTESIAN_POINT ( 'NONE',  ( 34.28542361028948449, 108.1059200568371068, 1.103255912984089537 ) ) ;
#8477=ORIENTED_EDGE ( 'NONE', *, *, #13139, .T. ) ;
#8485=ADVANCED_FACE ( 'NONE', ( #2543 ), #13386, .T. ) ;
#8500=VECTOR ( 'NONE', #1011, 1000.000000000000000 ) ;
#8502=DIRECTION ( 'NONE',  ( 0.000000000000000000, 0.000000000000000000, -1.000000000000000000 ) ) ;
#8506=DIRECTION ( 'NONE',  ( 1.000000000000000000, 0.000000000000000000, 0.000000000000000000 ) ) ;
#8540=ORIENTED_EDGE ( 'NONE', *, *, #5677, .F. ) ;
#8549=CYLINDRICAL_SURFACE ( 'NONE', #2875, 4.999999999999998224 ) ;
#8557=ORIENTED_EDGE ( 'NONE', *, *, #3773, .T. ) ;
#8561=ORIENTED_EDGE ( 'NONE', *, *, #6019, .T. ) ;
#8569=DIRECTION ( 'NONE',  ( 1.000000000000000000, 2.775557561562892929E-15, 0.000000000000000000 ) ) ;
#8572=DIRECTION ( 'NONE',  ( 0.8907235428302465730, -0.4545454545454549189, 0.000000000000000000 ) ) ;
#8581=EDGE_LOOP ( 'NONE', ( #4631, #12750, #5682, #8157, #11335 ) ) ;
#8582=ORIENTED_EDGE ( 'NONE', *, *, #12359, .F. ) ;
#8591=ADVANCED_FACE ( 'NONE', ( #4404 ), #12988, .F. ) ;
#8592=FACE_OUTER_BOUND ( 'NONE', #12465, .T. ) ;
#8620=AXIS2_PLACEMENT_3D ( 'NONE', #2468, #11168, #1554 ) ;
#8646=DIRECTION ( 'NONE',  ( 0.000000000000000000, 0.000000000000000000, 1.000000000000000000 ) ) ;
#8647=VERTEX_POINT ( 'NONE', #10240 ) ;
#8648=CARTESIAN_POINT ( 'NONE',  ( -49.99999999999999289, 120.0000000000000142, 0.5000000000000000000 ) ) ;
#8652=VERTEX_POINT ( 'NONE', #12277 ) ;
#8653=DIRECTION ( 'NONE',  ( 1.000000000000000000, 0.000000000000000000, 0.000000000000000000 ) ) ;
#8655=CARTESIAN_POINT ( 'NONE',  ( 34.25812584745457912, 108.1980041606221334, -0.6234749816336034867 ) ) ;
#8657=CARTESIAN_POINT ( 'NONE',  ( 40.81228451836345528, 100.6358150620708329, 0.5000000000000000000 ) ) ;
#8660=LINE ( 'NONE', #1102, #2429 ) ;
#8666=EDGE_CURVE ( 'NONE', #5463, #9616, #7136, .T. ) ;
#8671=CARTESIAN_POINT ( 'NONE',  ( -25.00000000000000355, 120.0000000000000142, -2.499999999999998668 ) ) ;
#8672=DIRECTION ( 'NONE',  ( 1.086108692045681373E-16, -1.448144922727572616E-16, 1.000000000000000000 ) ) ;
#8675=ORIENTED_EDGE ( 'NONE', *, *, #11665, .T. ) ;
#8678=EDGE_CURVE ( 'NONE', #10096, #1833, #650, .T. ) ;
#8683=AXIS2_PLACEMENT_3D ( 'NONE', #7869, #6054, #596 ) ;
#8686=CARTESIAN_POINT ( 'NONE',  ( 40.81228451836345528, 100.6358150620708329, -0.5000000000000000000 ) ) ;
#8693=AXIS2_PLACEMENT_3D ( 'NONE', #4242, #3196, #7474 ) ;
#8694=DIRECTION ( 'NONE',  ( 1.000000000000000000, 0.000000000000000000, -0.000000000000000000 ) ) ;
#8704=FACE_OUTER_BOUND ( 'NONE', #13205, .T. ) ;
#8705=LINE ( 'NONE', #11867, #13091 ) ;
#8711=CIRCLE ( 'NONE', #2685, 4.999999999999997335 ) ;
#8718=CARTESIAN_POINT ( 'NONE',  ( 34.28525802518650778, 108.1064455385057812, -1.101804919165826124 ) ) ;
#8719=CARTESIAN_POINT ( 'NONE',  ( 36.50000000000000711, 113.0000000000000142, -7.500000000000000000 ) ) ;
#8721=CARTESIAN_POINT ( 'NONE',  ( 40.68412312724077395, 100.6732077982500897, 1.167148848990505750 ) ) ;
#8723=AXIS2_PLACEMENT_3D ( 'NONE', #5499, #1359, #7669 ) ;
#8725=DIRECTION ( 'NONE',  ( -0.000000000000000000, -0.000000000000000000, -1.000000000000000000 ) ) ;
#8728=AXIS2_PLACEMENT_3D ( 'NONE', #13783, #2096, #12575 ) ;
#8734=B_SPLINE_CURVE_WITH_KNOTS ( 'NONE', 3,
 ( #8657, #1173, #6693, #1366, #8721, #11814, #5428, #7601, #2205, #2280, #8795, #3461, #6492, #11885, #4589, #10820 ),
 .UNSPECIFIED., .F., .F.,
 ( 4, 2, 2, 2, 2, 2, 2, 4 ),
 ( 1.967444805628318194E-07, 0.0004077652619395025148, 0.0008153337793984422781, 0.001630470814316321588, 0.002038039331775261514, 0.002445607849234201006, 0.002853176366693140498, 0.003260744884152080424 ),
 .UNSPECIFIED. ) ;
#8735=CIRCLE ( 'NONE', #9865, 4.999999999999998224 ) ;
#8758=CARTESIAN_POINT ( 'NONE',  ( -40.81228451836347659, 100.6358150620708471, 0.5000000000000000000 ) ) ;
#8763=ORIENTED_EDGE ( 'NONE', *, *, #7360, .T. ) ;
#8764=AXIS2_PLACEMENT_3D ( 'NONE', #13302, #2752, #6745 ) ;
#8765=DIRECTION ( 'NONE',  ( 0.000000000000000000, 0.000000000000000000, 1.000000000000000000 ) ) ;
#8771=LINE ( 'NONE', #6401, #9170 ) ;
#8773=CYLINDRICAL_SURFACE ( 'NONE', #10055, 27.49999999999999289 ) ;
#8778=CYLINDRICAL_SURFACE ( 'NONE', #9713, 69.99999999999998579 ) ;
#8782=ORIENTED_EDGE ( 'NONE', *, *, #11673, .T. ) ;
#8795=CARTESIAN_POINT ( 'NONE',  ( 39.64259366921353944, 101.1295926276828538, 2.298140577494254266 ) ) ;
#8797=AXIS2_PLACEMENT_3D ( 'NONE', #12407, #10160, #8968 ) ;
#8800=ORIENTED_EDGE ( 'NONE', *, *, #3955, .T. ) ;
#8801=DIRECTION ( 'NONE',  ( 0.000000000000000000, 0.000000000000000000, -1.000000000000000000 ) ) ;
#8804=CARTESIAN_POINT ( 'NONE',  ( -52.50000000000000000, 120.0000000000000142, 7.500000000000000000 ) ) ;
#8809=DIRECTION ( 'NONE',  ( 1.000000000000000000, 0.000000000000000000, 0.000000000000000000 ) ) ;
#8824=DIRECTION ( 'NONE',  ( 1.000000000000000000, 0.000000000000000000, 0.000000000000000000 ) ) ;
#8837=ORIENTED_EDGE ( 'NONE', *, *, #9875, .F. ) ;
#8857=EDGE_CURVE ( 'NONE', #3876, #2956, #3534, .T. ) ;
#8861=ORIENTED_EDGE ( 'NONE', *, *, #5868, .F. ) ;
#8864=ORIENTED_EDGE ( 'NONE', *, *, #9547, .F. ) ;
#8868=DIRECTION ( 'NONE',  ( -0.000000000000000000, -0.000000000000000000, -1.000000000000000000 ) ) ;
#8870=CARTESIAN_POINT ( 'NONE',  ( 34.46489652880494248, 107.6161854625081276, -1.920135329999817175 ) ) ;
#8880=DIRECTION ( 'NONE',  ( -1.000000000000000000, 0.000000000000000000, 0.000000000000000000 ) ) ;
#8887=CARTESIAN_POINT ( 'NONE',  ( -39.64464840659820766, 101.1283747906781088, 2.297097423097428592 ) ) ;
#8889=CARTESIAN_POINT ( 'NONE',  ( 37.49999999999999289, 120.0000000000000142, 2.499999999999999556 ) ) ;
#8890=VERTEX_POINT ( 'NONE', #5585 ) ;
#8895=LINE ( 'NONE', #1530, #4728 ) ;
#8897=ORIENTED_EDGE ( 'NONE', *, *, #12026, .F. ) ;
#8898=DIRECTION ( 'NONE',  ( -1.000000000000000000, 0.000000000000000000, 0.000000000000000000 ) ) ;
#8921=CYLINDRICAL_SURFACE ( 'NONE', #781, 12.49999999999999289 ) ;
#8922=LINE ( 'NONE', #2464, #12527 ) ;
#8927=CARTESIAN_POINT ( 'NONE',  ( 35.06230589874905945, 106.5835921350012683, 2.499999999999999556 ) ) ;
#8929=FACE_OUTER_BOUND ( 'NONE', #3538, .T. ) ;
#8935=VERTEX_POINT ( 'NONE', #13198 ) ;
#8942=EDGE_LOOP ( 'NONE', ( #7550, #8477, #3859 ) ) ;
#8947=DIRECTION ( 'NONE',  ( 0.000000000000000000, 0.000000000000000000, 1.000000000000000000 ) ) ;
#8949=CARTESIAN_POINT ( 'NONE',  ( -25.00000000000000355, 120.0000000000000142, 2.499999999999999556 ) ) ;
#8966=DIRECTION ( 'NONE',  ( -1.000000000000000000, 0.000000000000000000, 0.000000000000000000 ) ) ;
#8967=ADVANCED_FACE ( 'NONE', ( #4833 ), #2208, .F. ) ;
#8968=DIRECTION ( 'NONE',  ( 0.7999999999999996003, 0.6000000000000007550, 0.000000000000000000 ) ) ;
#8969=AXIS2_PLACEMENT_3D ( 'NONE', #2162, #4617, #8898 ) ;
#8988=FACE_OUTER_BOUND ( 'NONE', #7343, .T. ) ;
#8991=ORIENTED_EDGE ( 'NONE', *, *, #9712, .T. ) ;
#8995=SPHERICAL_SURFACE ( 'NONE', #1877, 5.000000000000000000 ) ;
#9002=ORIENTED_EDGE ( 'NONE', *, *, #12359, .T. ) ;
#9003=VERTEX_POINT ( 'NONE', #9171 ) ;
#9005=VERTEX_POINT ( 'NONE', #8889 ) ;
#9039=ORIENTED_EDGE ( 'NONE', *, *, #2065, .T. ) ;
#9041=AXIS2_PLACEMENT_3D ( 'NONE', #11643, #10716, #10591 ) ;
#9048=CARTESIAN_POINT ( 'NONE',  ( 42.16244658108818300, 105.4500712252157797, -2.499999999999999556 ) ) ;
#9053=AXIS2_PLACEMENT_3D ( 'NONE', #273, #2425, #6706 ) ;
#9079=CARTESIAN_POINT ( 'NONE',  ( 30.68181818181819054, 131.1340442853780530, -2.499999999999998668 ) ) ;
#9085=ORIENTED_EDGE ( 'NONE', *, *, #3096, .T. ) ;
#9090=EDGE_CURVE ( 'NONE', #8935, #8890, #662, .T. ) ;
#9099=DIRECTION ( 'NONE',  ( 0.6000000000000001998, 0.7999999999999998224, -0.000000000000000000 ) ) ;
#9104=EDGE_CURVE ( 'NONE', #780, #214, #4047, .T. ) ;
#9109=DIRECTION ( 'NONE',  ( 1.000000000000000000, 0.000000000000000000, 0.000000000000000000 ) ) ;
#9115=ORIENTED_EDGE ( 'NONE', *, *, #7123, .F. ) ;
#9118=EDGE_CURVE ( 'NONE', #9823, #7882, #10061, .T. ) ;
#9127=DIRECTION ( 'NONE',  ( -1.000000000000000000, 0.000000000000000000, 0.000000000000000000 ) ) ;
#9131=SURFACE_STYLE_FILL_AREA ( #2679 ) ;
#9138=ORIENTED_EDGE ( 'NONE', *, *, #2398, .F. ) ;
#9139=VERTEX_POINT ( 'NONE', #2859 ) ;
#9141=ORIENTED_EDGE ( 'NONE', *, *, #10380, .F. ) ;
#9144=CARTESIAN_POINT ( 'NONE',  ( -39.06230589874905235, 109.5835921350012825, 2.499999999999999556 ) ) ;
#9151=DIRECTION ( 'NONE',  ( 0.000000000000000000, 0.000000000000000000, 1.000000000000000000 ) ) ;
#9152=CARTESIAN_POINT ( 'NONE',  ( -38.89115197531750567, 101.6687180808697519, -2.500000000000000000 ) ) ;
#9153=DIRECTION ( 'NONE',  ( -0.8907235428302473501, 0.4545454545454531425, 0.000000000000000000 ) ) ;
#9160=ORIENTED_EDGE ( 'NONE', *, *, #1540, .F. ) ;
#9168=CARTESIAN_POINT ( 'NONE',  ( -40.74280923682185573, 100.6542365527006098, 1.046903941091061885 ) ) ;
#9170=VECTOR ( 'NONE', #5342, 1000.000000000000000 ) ;
#9171=CARTESIAN_POINT ( 'NONE',  ( -31.81818181818181657, 133.3608531424536920, 0.5000000000000000000 ) ) ;
#9183=CARTESIAN_POINT ( 'NONE',  ( 37.50000000000002132, 144.4948974278317735, -2.499999999999998668 ) ) ;
#9188=AXIS2_PLACEMENT_3D ( 'NONE', #11074, #5743, #5820 ) ;
#9198=EDGE_CURVE ( 'NONE', #11053, #6878, #8660, .T. ) ;
#9200=FILL_AREA_STYLE_COLOUR ( '', #2356 ) ;
#9201=EDGE_CURVE ( 'NONE', #2829, #9570, #2345, .T. ) ;
#9218=CIRCLE ( 'NONE', #11444, 2.000000000000003997 ) ;
#9226=DIRECTION ( 'NONE',  ( 1.000000000000000000, 3.581364595565021862E-15, 0.000000000000000000 ) ) ;
#9228=DIRECTION ( 'NONE',  ( -0.000000000000000000, -0.000000000000000000, -1.000000000000000000 ) ) ;
#9230=DIRECTION ( 'NONE',  ( -0.000000000000000000, -0.000000000000000000, 1.000000000000000000 ) ) ;
#9232=TOROIDAL_SURFACE ( 'NONE', #3160, 77.49999999999998579, 5.000000000000000000 ) ;
#9233=ORIENTED_EDGE ( 'NONE', *, *, #12026, .T. ) ;
#9246=ORIENTED_EDGE ( 'NONE', *, *, #5666, .T. ) ;
#9252=CARTESIAN_POINT ( 'NONE',  ( 34.63116476221791373, 107.2647840444379028, 2.216888271186473691 ) ) ;
#9256=EDGE_CURVE ( 'NONE', #13223, #8652, #1104, .T. ) ;
#9257=DIRECTION ( 'NONE',  ( 0.000000000000000000, 0.000000000000000000, -1.000000000000000000 ) ) ;
#9263=DIRECTION ( 'NONE',  ( 0.8035603370713739757, -0.5952233065713573579, 0.000000000000000000 ) ) ;
#9265=FACE_OUTER_BOUND ( 'NONE', #303, .T. ) ;
#9271=EDGE_CURVE ( 'NONE', #9823, #10096, #13459, .T. ) ;
#9276=ORIENTED_EDGE ( 'NONE', *, *, #6966, .T. ) ;
#9281=ADVANCED_FACE ( 'NONE', ( #12898 ), #1532, .F. ) ;
#9285=DIRECTION ( 'NONE',  ( 0.000000000000000000, 0.000000000000000000, 1.000000000000000000 ) ) ;
#9288=CIRCLE ( 'NONE', #11739, 4.999999999999997335 ) ;
#9292=DIRECTION ( 'NONE',  ( 0.7627754036039218200, 0.6466635011015190448, 0.000000000000000000 ) ) ;
#9294=DIRECTION ( 'NONE',  ( 0.000000000000000000, 0.000000000000000000, 1.000000000000000000 ) ) ;
#9298=ORIENTED_EDGE ( 'NONE', *, *, #8666, .T. ) ;
#9307=CYLINDRICAL_SURFACE ( 'NONE', #5945, 4.999999999999997335 ) ;
#9312=DIRECTION ( 'NONE',  ( 1.000000000000000000, 1.810146235801886110E-15, 0.000000000000000000 ) ) ;
#9316=ORIENTED_EDGE ( 'NONE', *, *, #12876, .T. ) ;
#9324=CARTESIAN_POINT ( 'NONE',  ( -45.97632359910779343, 102.2167537197081799, -2.499999999999998668 ) ) ;
#9342=DIRECTION ( 'NONE',  ( 0.6000000000000001998, -0.7999999999999999334, 0.000000000000000000 ) ) ;
#9353=ADVANCED_FACE ( 'NONE', ( #12251 ), #2496, .T. ) ;
#9355=ORIENTED_EDGE ( 'NONE', *, *, #12336, .F. ) ;
#9374=EDGE_LOOP ( 'NONE', ( #5022, #5199, #9736, #1310 ) ) ;
#9377=AXIS2_PLACEMENT_3D ( 'NONE', #11626, #5110, #11566 ) ;
#9396=FACE_OUTER_BOUND ( 'NONE', #5130, .T. ) ;
#9403=VECTOR ( 'NONE', #6344, 1000.000000000000000 ) ;
#9404=ORIENTED_EDGE ( 'NONE', *, *, #9271, .F. ) ;
#9422=CARTESIAN_POINT ( 'NONE',  ( -39.06230589874905235, 109.5835921350012683, -2.499999999999998668 ) ) ;
#9425=DIRECTION ( 'NONE',  ( 1.000000000000000000, 0.000000000000000000, 0.000000000000000000 ) ) ;
#9428=AXIS2_PLACEMENT_3D ( 'NONE', #3885, #1498, #13467 ) ;
#9431=DIRECTION ( 'NONE',  ( 1.000000000000000000, -1.665334536937735599E-15, 0.000000000000000000 ) ) ;
#9435=CIRCLE ( 'NONE', #2249, 12.49999999999998757 ) ;
#9436=EDGE_CURVE ( 'NONE', #9003, #4466, #1313, .T. ) ;
#9437=CARTESIAN_POINT ( 'NONE',  ( -52.50000000000000000, 120.0000000000000142, 2.499999999999999556 ) ) ;
#9438=COLOUR_RGB ( '', 0.66274510, 0.83137255, 0.94901961) ;
#9459=VERTEX_POINT ( 'NONE', #9759 ) ;
#9462=ORIENTED_EDGE ( 'NONE', *, *, #11823, .F. ) ;
#9464=CARTESIAN_POINT ( 'NONE',  ( 34.73643445648811934, 107.0738672501280462, 2.329477027598938044 ) ) ;
#9467=EDGE_CURVE ( 'NONE', #2436, #11706, #8771, .T. ) ;
#9473=ORIENTED_EDGE ( 'NONE', *, *, #874, .F. ) ;
#9476=ORIENTED_EDGE ( 'NONE', *, *, #5265, .T. ) ;
#9477=CARTESIAN_POINT ( 'NONE',  ( 35.04450421339217314, 112.5597086678580609, -2.499999999999998668 ) ) ;
#9490=FACE_OUTER_BOUND ( 'NONE', #11468, .T. ) ;
#9494=CARTESIAN_POINT ( 'NONE',  ( 34.25812584745457201, 108.1980041606221050, 0.5000000000000000000 ) ) ;
#9500=AXIS2_PLACEMENT_3D ( 'NONE', #10414, #2059, #13876 ) ;
#9504=EDGE_LOOP ( 'NONE', ( #12058, #12434, #8379, #9138, #4077, #2747 ) ) ;
#9509=CARTESIAN_POINT ( 'NONE',  ( 36.36363636363638108, 142.2680885707561629, 2.500000000000000000 ) ) ;
#9510=LINE ( 'NONE', #8453, #5818 ) ;
#9516=VERTEX_POINT ( 'NONE', #4415 ) ;
#9532=DIRECTION ( 'NONE',  ( 0.000000000000000000, -1.000000000000000000, 0.000000000000000000 ) ) ;
#9534=EDGE_LOOP ( 'NONE', ( #2002, #10233, #8156 ) ) ;
#9542=ORIENTED_EDGE ( 'NONE', *, *, #9635, .T. ) ;
#9547=EDGE_CURVE ( 'NONE', #9003, #2436, #1544, .T. ) ;
#9551=CARTESIAN_POINT ( 'NONE',  ( -25.00000000000000355, 120.0000000000000142, -0.5000000000000000000 ) ) ;
#9552=VERTEX_POINT ( 'NONE', #1003 ) ;
#9562=EDGE_CURVE ( 'NONE', #1278, #5368, #3038, .T. ) ;
#9568=ORIENTED_EDGE ( 'NONE', *, *, #10142, .F. ) ;
#9570=VERTEX_POINT ( 'NONE', #3951 ) ;
#9575=DIRECTION ( 'NONE',  ( 0.6000000000000001998, -0.7999999999999998224, -0.000000000000000000 ) ) ;
#9582=DIRECTION ( 'NONE',  ( 1.000000000000000000, 0.000000000000000000, 0.000000000000000000 ) ) ;
#9588=DIRECTION ( 'NONE',  ( 1.000000000000000000, 0.000000000000000000, 0.000000000000000000 ) ) ;
#9600=ADVANCED_FACE ( 'NONE', ( #9490 ), #3162, .T. ) ;
#9616=VERTEX_POINT ( 'NONE', #10665 ) ;
#9623=CARTESIAN_POINT ( 'NONE',  ( -25.00000000000000355, 120.0000000000000142, 7.500000000000000000 ) ) ;
#9630=CIRCLE ( 'NONE', #11420, 24.99999999999998934 ) ;
#9635=EDGE_CURVE ( 'NONE', #2097, #7028, #7153, .T. ) ;
#9637=ORIENTED_EDGE ( 'NONE', *, *, #3002, .F. ) ;
#9640=CIRCLE ( 'NONE', #13503, 12.49999999999999289 ) ;
#9648=DIRECTION ( 'NONE',  ( 1.000000000000000000, 3.532527805625498693E-15, 0.000000000000000000 ) ) ;
#9650=DIRECTION ( 'NONE',  ( 0.000000000000000000, 0.000000000000000000, 1.000000000000000000 ) ) ;
#9651=MECHANICAL_DESIGN_GEOMETRIC_PRESENTATION_REPRESENTATION('',(#2476),#10757);
#9659=DIRECTION ( 'NONE',  ( 1.000000000000000000, 0.000000000000000000, 0.000000000000000000 ) ) ;
#9670=AXIS2_PLACEMENT_3D ( 'NONE', #9961, #10477, #330 ) ;
#9675=CARTESIAN_POINT ( 'NONE',  ( 40.81228451836656035, 100.6358150620699803, -0.7758357214534923330 ) ) ;
#9680=ORIENTED_EDGE ( 'NONE', *, *, #9753, .T. ) ;
#9684=VERTEX_POINT ( 'NONE', #2312 ) ;
#9686=CARTESIAN_POINT ( 'NONE',  ( 34.25812584745457201, 108.1980041606221050, 0.000000000000000000 ) ) ;
#9707=ORIENTED_EDGE ( 'NONE', *, *, #5095, .T. ) ;
#9710=DIRECTION ( 'NONE',  ( 0.000000000000000000, 0.000000000000000000, 1.000000000000000000 ) ) ;
#9712=EDGE_CURVE ( 'NONE', #6075, #973, #10074, .T. ) ;
#9713=AXIS2_PLACEMENT_3D ( 'NONE', #3507, #10675, #1085 ) ;
#9716=CARTESIAN_POINT ( 'NONE',  ( 25.00000000000000355, 120.0000000000000142, 2.500000000000000000 ) ) ;
#9717=CARTESIAN_POINT ( 'NONE',  ( 0.000000000000000000, 71.01020514433645303, -2.499999999999998668 ) ) ;
#9731=DIRECTION ( 'NONE',  ( -1.000000000000000000, 0.000000000000000000, 0.000000000000000000 ) ) ;
#9733=AXIS2_PLACEMENT_3D ( 'NONE', #3384, #2271, #1430 ) ;
#9736=ORIENTED_EDGE ( 'NONE', *, *, #10455, .F. ) ;
#9740=ORIENTED_EDGE ( 'NONE', *, *, #7100, .F. ) ;
#9744=CARTESIAN_POINT ( 'NONE',  ( -34.50158885938634512, 107.5319404580926204, -2.003700325319502262 ) ) ;
#9749=EDGE_LOOP ( 'NONE', ( #7608, #5774, #10976, #5321, #13659 ) ) ;
#9752=CIRCLE ( 'NONE', #362, 69.99999999999998579 ) ;
#9753=EDGE_CURVE ( 'NONE', #973, #2515, #4231, .T. ) ;
#9754=FACE_OUTER_BOUND ( 'NONE', #281, .T. ) ;
#9759=CARTESIAN_POINT ( 'NONE',  ( 31.81818181818183433, 133.3608531424536920, 0.5000000000000000000 ) ) ;
#9761=( GEOMETRIC_REPRESENTATION_CONTEXT ( 3 ) GLOBAL_UNCERTAINTY_ASSIGNED_CONTEXT ( ( #698 ) ) GLOBAL_UNIT_ASSIGNED_CONTEXT ( ( #1042, #12966, #13834 ) ) REPRESENTATION_CONTEXT ( 'NONE', 'WORKASPACE' ) );
#9763=CIRCLE ( 'NONE', #7515, 17.49999999999999289 ) ;
#9772=EDGE_CURVE ( 'NONE', #1557, #4611, #3552, .T. ) ;
#9780=ADVANCED_FACE ( 'NONE', ( #9754 ), #2455, .T. ) ;
#9788=DIRECTION ( 'NONE',  ( 1.000000000000000000, 0.000000000000000000, 0.000000000000000000 ) ) ;
#9790=CARTESIAN_POINT ( 'NONE',  ( 25.00000000000000355, 120.0000000000000142, -7.500000000000000000 ) ) ;
#9795=ORIENTED_EDGE ( 'NONE', *, *, #1370, .T. ) ;
#9798=LINE ( 'NONE', #6638, #10407 ) ;
#9802=ORIENTED_EDGE ( 'NONE', *, *, #9090, .T. ) ;
#9805=ADVANCED_FACE ( 'NONE', ( #12142 ), #3568, .F. ) ;
#9808=ORIENTED_EDGE ( 'NONE', *, *, #6787, .F. ) ;
#9814=DIRECTION ( 'NONE',  ( 1.000000000000000000, -2.775557561562892929E-15, 0.000000000000000000 ) ) ;
#9820=ORIENTED_EDGE ( 'NONE', *, *, #3508, .T. ) ;
#9823=VERTEX_POINT ( 'NONE', #7856 ) ;
#9830=EDGE_CURVE ( 'NONE', #2762, #7525, #11957, .T. ) ;
#9850=CYLINDRICAL_SURFACE ( 'NONE', #7614, 4.999999999999993783 ) ;
#9858=AXIS2_PLACEMENT_3D ( 'NONE', #7889, #10272, #4945 ) ;
#9862=ORIENTED_EDGE ( 'NONE', *, *, #13760, .F. ) ;
#9865=AXIS2_PLACEMENT_3D ( 'NONE', #1853, #814, #8309 ) ;
#9875=EDGE_CURVE ( 'NONE', #5368, #11053, #4330, .T. ) ;
#9877=ADVANCED_FACE ( 'NONE', ( #8988 ), #1884, .T. ) ;
#9879=APPLICATION_CONTEXT ( 'automotive_design' ) ;
#9880=VERTEX_POINT ( 'NONE', #13295 ) ;
#9882=CIRCLE ( 'NONE', #11446, 5.000000000000004441 ) ;
#9891=DIRECTION ( 'NONE',  ( -1.000000000000000000, 0.000000000000000000, 0.000000000000000000 ) ) ;
#9895=ORIENTED_EDGE ( 'NONE', *, *, #8176, .F. ) ;
#9898=AXIS2_PLACEMENT_3D ( 'NONE', #7384, #7251, #1928 ) ;
#9900=ORIENTED_EDGE ( 'NONE', *, *, #6429, .T. ) ;
#9904=DIRECTION ( 'NONE',  ( -1.000000000000000000, 0.000000000000000000, 0.000000000000000000 ) ) ;
#9907=CARTESIAN_POINT ( 'NONE',  ( 0.000000000000000000, 71.01020514433645303, 7.500000000000000000 ) ) ;
#9916=AXIS2_PLACEMENT_3D ( 'NONE', #895, #7266, #9312 ) ;
#9917=ORIENTED_EDGE ( 'NONE', *, *, #2590, .T. ) ;
#9920=DIRECTION ( 'NONE',  ( -0.000000000000000000, -0.000000000000000000, -1.000000000000000000 ) ) ;
#9922=CARTESIAN_POINT ( 'NONE',  ( 42.49999999999999289, 120.0000000000000142, 7.500000000000000000 ) ) ;
#9928=CARTESIAN_POINT ( 'NONE',  ( -32.72727272727271952, 135.1423002281141805, 0.5000000000000000000 ) ) ;
#9932=EDGE_CURVE ( 'NONE', #8652, #7028, #11060, .T. ) ;
#9943=AXIS2_PLACEMENT_3D ( 'NONE', #2745, #5684, #1619 ) ;
#9944=ORIENTED_EDGE ( 'NONE', *, *, #7288, .F. ) ;
#9955=FACE_OUTER_BOUND ( 'NONE', #7929, .T. ) ;
#9961=CARTESIAN_POINT ( 'NONE',  ( 32.72727272727274084, 135.1423002281141805, 0.5000000000000000000 ) ) ;
#9971=DIRECTION ( 'NONE',  ( -0.000000000000000000, -0.000000000000000000, -1.000000000000000000 ) ) ;
#9983=AXIS2_PLACEMENT_3D ( 'NONE', #9551, #8154, #11372 ) ;
#9994=AXIS2_PLACEMENT_3D ( 'NONE', #11271, #1666, #12467 ) ;
#9999=LINE ( 'NONE', #8719, #2467 ) ;
#10000=CARTESIAN_POINT ( 'NONE',  ( 25.00000000000000355, 120.0000000000000142, 0.5000000000000000000 ) ) ;
#10003=CIRCLE ( 'NONE', #381, 82.49999999999998579 ) ;
#10012=DIRECTION ( 'NONE',  ( -0.000000000000000000, -0.000000000000000000, -1.000000000000000000 ) ) ;
#10022=( NAMED_UNIT ( * ) PLANE_ANGLE_UNIT ( ) SI_UNIT ( $, .RADIAN. ) );
#10043=LINE ( 'NONE', #592, #435 ) ;
#10050=ORIENTED_EDGE ( 'NONE', *, *, #7773, .T. ) ;
#10051=AXIS2_PLACEMENT_3D ( 'NONE', #11983, #3357, #9891 ) ;
#10053=EDGE_LOOP ( 'NONE', ( #1726, #9141, #6153, #1660, #12198, #9160 ) ) ;
#10055=AXIS2_PLACEMENT_3D ( 'NONE', #3500, #12071, #9904 ) ;
#10061=CIRCLE ( 'NONE', #3781, 5.000000000000005329 ) ;
#10068=DIRECTION ( 'NONE',  ( -1.000000000000000000, 0.000000000000000000, 0.000000000000000000 ) ) ;
#10074=CIRCLE ( 'NONE', #2435, 5.000000000000000888 ) ;
#10081=ORIENTED_EDGE ( 'NONE', *, *, #13335, .F. ) ;
#10085=CARTESIAN_POINT ( 'NONE',  ( -39.10224891377573897, 101.4936815461678208, 2.486392430613896032 ) ) ;
#10090=VERTEX_POINT ( 'NONE', #7423 ) ;
#10096=VERTEX_POINT ( 'NONE', #2574 ) ;
#10111=DIRECTION ( 'NONE',  ( 1.000000000000000000, 0.000000000000000000, 0.000000000000000000 ) ) ;
#10115=CIRCLE ( 'NONE', #7421, 16.99999999999998934 ) ;
#10116=FACE_OUTER_BOUND ( 'NONE', #1222, .T. ) ;
#10126=ORIENTED_EDGE ( 'NONE', *, *, #13221, .F. ) ;
#10134=DIRECTION ( 'NONE',  ( 1.000000000000000000, -3.851859888774468203E-30, 1.387778780781445676E-15 ) ) ;
#10135=VERTEX_POINT ( 'NONE', #5725 ) ;
#10142=EDGE_CURVE ( 'NONE', #3010, #1557, #11131, .T. ) ;
#10144=DIRECTION ( 'NONE',  ( -0.000000000000000000, -0.000000000000000000, -1.000000000000000000 ) ) ;
#10154=DIRECTION ( 'NONE',  ( 0.000000000000000000, 0.000000000000000000, 1.000000000000000000 ) ) ;
#10160=DIRECTION ( 'NONE',  ( 0.6000000000000006439, -0.7999999999999996003, 0.000000000000000000 ) ) ;
#10168=FILL_AREA_STYLE_COLOUR ( '', #9438 ) ;
#10175=ORIENTED_EDGE ( 'NONE', *, *, #5565, .T. ) ;
#10182=LINE ( 'NONE', #727, #3322 ) ;
#10185=CARTESIAN_POINT ( 'NONE',  ( -39.06230589874905235, 109.5835921350012825, -2.499999999999999556 ) ) ;
#10207=CARTESIAN_POINT ( 'NONE',  ( 0.000000000000000000, 71.01020514433645303, -0.5000000000000000000 ) ) ;
#10233=ORIENTED_EDGE ( 'NONE', *, *, #2135, .T. ) ;
#10238=CARTESIAN_POINT ( 'NONE',  ( -34.78790783510986984, 106.9804631782722169, 2.384639261440467006 ) ) ;
#10240=CARTESIAN_POINT ( 'NONE',  ( -36.36363636363635976, 142.2680885707561629, -0.5000000000000000000 ) ) ;
#10243=EDGE_CURVE ( 'NONE', #7167, #6716, #4552, .T. ) ;
#10244=ORIENTED_EDGE ( 'NONE', *, *, #12082, .T. ) ;
#10260=EDGE_LOOP ( 'NONE', ( #1385, #3271, #7592, #6364, #3533 ) ) ;
#10263=B_SPLINE_CURVE_WITH_KNOTS ( 'NONE', 3,
 ( #995, #1065, #10780, #6318, #5259, #5328, #5458, #9744, #4402, #3354, #7635, #11910, #2300, #512, #3484, #2663, #1468, #436 ),
 .UNSPECIFIED., .F., .F.,
 ( 4, 2, 2, 2, 2, 2, 2, 2, 4 ),
 ( 2.478944061727388434E-07, 0.0003651306916264178350, 0.0007300134888466628617, 0.001094896286066908159, 0.001459779083287153023, 0.001824661880507398104, 0.002189544677727643836, 0.002554427474947888917, 0.002919310272168133130 ),
 .UNSPECIFIED. ) ;
#10271=CARTESIAN_POINT ( 'NONE',  ( -25.00000000000000355, 120.0000000000000142, -2.499999999999998668 ) ) ;
#10272=DIRECTION ( 'NONE',  ( 0.000000000000000000, -1.000000000000000000, 0.000000000000000000 ) ) ;
#10275=CARTESIAN_POINT ( 'NONE',  ( 0.000000000000000000, 71.01020514433645303, 2.499999999999999556 ) ) ;
#10292=ADVANCED_FACE ( 'NONE', ( #12328 ), #9307, .T. ) ;
#10297=VECTOR ( 'NONE', #10807, 1000.000000000000000 ) ;
#10313=CIRCLE ( 'NONE', #900, 4.999999999999998224 ) ;
#10315=AXIS2_PLACEMENT_3D ( 'NONE', #2203, #6490, #11883 ) ;
#10328=CIRCLE ( 'NONE', #13729, 22.99999999999999645 ) ;
#10332=ORIENTED_EDGE ( 'NONE', *, *, #3701, .F. ) ;
#10334=ORIENTED_EDGE ( 'NONE', *, *, #13335, .T. ) ;
#10339=DIRECTION ( 'NONE',  ( -0.000000000000000000, -0.000000000000000000, -1.000000000000000000 ) ) ;
#10341=DIRECTION ( 'NONE',  ( 1.000000000000000000, 0.000000000000000000, 0.000000000000000000 ) ) ;
#10348=CARTESIAN_POINT ( 'NONE',  ( 42.16244658108818300, 105.4500712252157655, -2.499999999999999556 ) ) ;
#10350=VERTEX_POINT ( 'NONE', #6224 ) ;
#10352=ORIENTED_EDGE ( 'NONE', *, *, #13161, .T. ) ;
#10371=CARTESIAN_POINT ( 'NONE',  ( 34.37593967123855521, 107.8393652239837195, 1.644494279733350162 ) ) ;
#10378=ADVANCED_FACE ( 'NONE', ( #12678 ), #578, .T. ) ;
#10379=ORIENTED_EDGE ( 'NONE', *, *, #8413, .T. ) ;
#10380=EDGE_CURVE ( 'NONE', #2194, #5379, #1896, .T. ) ;
#10392=AXIS2_PLACEMENT_3D ( 'NONE', #4357, #4421, #7519 ) ;
#10405=DIRECTION ( 'NONE',  ( 0.000000000000000000, 0.000000000000000000, 1.000000000000000000 ) ) ;
#10407=VECTOR ( 'NONE', #1450, 1000.000000000000000 ) ;
#10414=CARTESIAN_POINT ( 'NONE',  ( 0.000000000000000000, 71.01020514433645303, 0.5000000000000000000 ) ) ;
#10416=CARTESIAN_POINT ( 'NONE',  ( -25.00000000000000355, 120.0000000000000142, -0.5000000000000000000 ) ) ;
#10418=CIRCLE ( 'NONE', #6170, 17.49999999999999289 ) ;
#10436=AXIS2_PLACEMENT_3D ( 'NONE', #7698, #2368, #1319 ) ;
#10439=AXIS2_PLACEMENT_3D ( 'NONE', #7180, #13542, #13674 ) ;
#10446=ORIENTED_EDGE ( 'NONE', *, *, #12356, .F. ) ;
#10455=EDGE_CURVE ( 'NONE', #4214, #8450, #4234, .T. ) ;
#10472=FACE_OUTER_BOUND ( 'NONE', #6864, .T. ) ;
#10474=ADVANCED_FACE ( 'NONE', ( #3117 ), #6486, .T. ) ;
#10477=DIRECTION ( 'NONE',  ( -0.8907235428302473501, 0.4545454545454531425, 0.000000000000000000 ) ) ;
#10483=CARTESIAN_POINT ( 'NONE',  ( 25.00000000000000355, 120.0000000000000142, 2.499999999999999556 ) ) ;
#10487=AXIS2_PLACEMENT_3D ( 'NONE', #3008, #9532, #9257 ) ;
#10493=EDGE_CURVE ( 'NONE', #2984, #7882, #2109, .T. ) ;
#10496=AXIS2_PLACEMENT_3D ( 'NONE', #5506, #11816, #9582 ) ;
#10502=CARTESIAN_POINT ( 'NONE',  ( 34.25812584745450096, 108.1980041606223466, 0.6234894336158707251 ) ) ;
#10510=CARTESIAN_POINT ( 'NONE',  ( 0.000000000000000000, 71.01020514433645303, -7.500000000000000000 ) ) ;
#10513=EDGE_LOOP ( 'NONE', ( #8561, #3993, #12998, #8043 ) ) ;
#10527=ORIENTED_EDGE ( 'NONE', *, *, #13055, .F. ) ;
#10537=TOROIDAL_SURFACE ( 'NONE', #12799, 16.99999999999998934, 2.000000000000000000 ) ;
#10542=DIRECTION ( 'NONE',  ( 0.000000000000000000, 0.000000000000000000, 1.000000000000000000 ) ) ;
#10552=ORIENTED_EDGE ( 'NONE', *, *, #7222, .F. ) ;
#10556=CYLINDRICAL_SURFACE ( 'NONE', #12892, 24.99999999999998934 ) ;
#10569=EDGE_CURVE ( 'NONE', #6314, #7422, #5465, .T. ) ;
#10579=ORIENTED_EDGE ( 'NONE', *, *, #9562, .F. ) ;
#10588=CARTESIAN_POINT ( 'NONE',  ( 36.36363636363638108, 142.2680885707561629, 0.5000000000000000000 ) ) ;
#10591=DIRECTION ( 'NONE',  ( -0.4545454545454548634, 0.8907235428302464619, 0.000000000000000000 ) ) ;
#10595=ORIENTED_EDGE ( 'NONE', *, *, #13794, .F. ) ;
#10597=ORIENTED_EDGE ( 'NONE', *, *, #7805, .F. ) ;
#10601=DIRECTION ( 'NONE',  ( 0.000000000000000000, 0.000000000000000000, 1.000000000000000000 ) ) ;
#10602=DIRECTION ( 'NONE',  ( -1.000000000000000000, 0.000000000000000000, 0.000000000000000000 ) ) ;
#10631=ORIENTED_EDGE ( 'NONE', *, *, #3630, .T. ) ;
#10634=FACE_OUTER_BOUND ( 'NONE', #8258, .T. ) ;
#10639=AXIS2_PLACEMENT_3D ( 'NONE', #13859, #7638, #1068 ) ;
#10645=EDGE_CURVE ( 'NONE', #4466, #12157, #5705, .T. ) ;
#10646=CIRCLE ( 'NONE', #5718, 5.000000000000004441 ) ;
#10655=CARTESIAN_POINT ( 'NONE',  ( 40.33442208022854913, 100.7954446087837823, -1.738653613625530614 ) ) ;
#10665=CARTESIAN_POINT ( 'NONE',  ( 50.00000000000000000, 120.0000000000000142, -0.5000000000000000000 ) ) ;
#10672=CARTESIAN_POINT ( 'NONE',  ( -30.68181818181819054, 131.1340442853780814, 7.500000000000000000 ) ) ;
#10675=DIRECTION ( 'NONE',  ( -0.000000000000000000, -0.000000000000000000, -1.000000000000000000 ) ) ;
#10676=CARTESIAN_POINT ( 'NONE',  ( -25.00000000000000355, 120.0000000000000142, -2.500000000000000000 ) ) ;
#10677=CARTESIAN_POINT ( 'NONE',  ( -25.00000000000000355, 120.0000000000000142, 0.5000000000000000000 ) ) ;
#10682=DIRECTION ( 'NONE',  ( 1.000000000000000000, 0.000000000000000000, 0.000000000000000000 ) ) ;
#10686=CARTESIAN_POINT ( 'NONE',  ( -36.36363636363635976, 142.2680885707561629, 0.5000000000000000000 ) ) ;
#10689=CARTESIAN_POINT ( 'NONE',  ( 31.81818181818183433, 133.3608531424536920, 2.500000000000000000 ) ) ;
#10697=DIRECTION ( 'NONE',  ( 0.000000000000000000, 0.000000000000000000, 1.000000000000000000 ) ) ;
#10700=FACE_OUTER_BOUND ( 'NONE', #3804, .T. ) ;
#10704=ORIENTED_EDGE ( 'NONE', *, *, #5677, .T. ) ;
#10710=EDGE_CURVE ( 'NONE', #12810, #13223, #10418, .T. ) ;
#10712=EDGE_CURVE ( 'NONE', #3748, #5379, #2318, .T. ) ;
#10713=DIRECTION ( 'NONE',  ( 0.7999999999999999334, -0.6000000000000001998, 0.000000000000000000 ) ) ;
#10716=DIRECTION ( 'NONE',  ( 0.8907235428302465730, 0.4545454545454549189, 0.000000000000000000 ) ) ;
#10720=AXIS2_PLACEMENT_3D ( 'NONE', #4410, #8694, #3645 ) ;
#10730=DIRECTION ( 'NONE',  ( 0.7627754036039197105, 0.6466635011015212653, 0.000000000000000000 ) ) ;
#10734=CARTESIAN_POINT ( 'NONE',  ( 25.00000000000000355, 120.0000000000000142, 2.500000000000000000 ) ) ;
#10735=CARTESIAN_POINT ( 'NONE',  ( 41.99999999999999289, 120.0000000000000142, -2.500000000000000000 ) ) ;
#10736=CARTESIAN_POINT ( 'NONE',  ( 32.95454545454546036, 135.5876619995293026, 2.499999999999999556 ) ) ;
#10737=CIRCLE ( 'NONE', #4032, 72.49999999999998579 ) ;
#10748=CARTESIAN_POINT ( 'NONE',  ( 47.49999999999999289, 120.0000000000000142, 7.500000000000000000 ) ) ;
#10753=CARTESIAN_POINT ( 'NONE',  ( 34.78790783510986984, 106.9804631782721884, -2.384639261440465674 ) ) ;
#10757=( GEOMETRIC_REPRESENTATION_CONTEXT ( 3 ) GLOBAL_UNCERTAINTY_ASSIGNED_CONTEXT ( ( #6570 ) ) GLOBAL_UNIT_ASSIGNED_CONTEXT ( ( #12413, #10022, #6101 ) ) REPRESENTATION_CONTEXT ( 'NONE', 'WORKASPACE' ) );
#10771=CARTESIAN_POINT ( 'NONE',  ( -25.00000000000000355, 120.0000000000000142, 2.500000000000000000 ) ) ;
#10780=CARTESIAN_POINT ( 'NONE',  ( -34.92076574184287097, 106.7798134293913961, -2.447438947438305590 ) ) ;
#10786=EDGE_CURVE ( 'NONE', #4611, #13845, #2116, .T. ) ;
#10792=CARTESIAN_POINT ( 'NONE',  ( -25.00000000000000355, 120.0000000000000142, -2.499999999999998668 ) ) ;
#10797=AXIS2_PLACEMENT_3D ( 'NONE', #1602, #3841, #5887 ) ;
#10802=DIRECTION ( 'NONE',  ( -0.000000000000000000, -0.000000000000000000, -1.000000000000000000 ) ) ;
#10807=DIRECTION ( 'NONE',  ( -0.000000000000000000, -0.000000000000000000, -1.000000000000000000 ) ) ;
#10811=ORIENTED_EDGE ( 'NONE', *, *, #2592, .T. ) ;
#10814=DIRECTION ( 'NONE',  ( -0.000000000000000000, -0.000000000000000000, -1.000000000000000000 ) ) ;
#10819=CYLINDRICAL_SURFACE ( 'NONE', #13842, 4.999999999999997335 ) ;
#10820=CARTESIAN_POINT ( 'NONE',  ( 38.89115197531749857, 101.6687180808697377, 2.499999999999999556 ) ) ;
#10827=ORIENTED_EDGE ( 'NONE', *, *, #10786, .T. ) ;
#10835=CIRCLE ( 'NONE', #9733, 2.000000000000003997 ) ;
#10838=ORIENTED_EDGE ( 'NONE', *, *, #2749, .F. ) ;
#10841=ADVANCED_FACE ( 'NONE', ( #2067 ), #1021, .T. ) ;
#10842=ORIENTED_EDGE ( 'NONE', *, *, #7059, .F. ) ;
#10843=CARTESIAN_POINT ( 'NONE',  ( -35.04450421339218025, 112.5597086678580609, -2.499999999999998668 ) ) ;
#10848=CARTESIAN_POINT ( 'NONE',  ( 40.56568360645881910, 100.7114851384503851, -1.410085254968634239 ) ) ;
#10852=ORIENTED_EDGE ( 'NONE', *, *, #2575, .F. ) ;
#10854=VERTEX_POINT ( 'NONE', #1937 ) ;
#10878=CARTESIAN_POINT ( 'NONE',  ( -37.50000000000002132, 144.4948974278317735, 7.500000000000000000 ) ) ;
#10924=AXIS2_PLACEMENT_3D ( 'NONE', #1525, #11211, #9109 ) ;
#10930=DIRECTION ( 'NONE',  ( 0.000000000000000000, 0.000000000000000000, 1.000000000000000000 ) ) ;
#10931=DIRECTION ( 'NONE',  ( 0.000000000000000000, 0.000000000000000000, 1.000000000000000000 ) ) ;
#10940=DIRECTION ( 'NONE',  ( 0.000000000000000000, 0.000000000000000000, 1.000000000000000000 ) ) ;
#10965=CIRCLE ( 'NONE', #13016, 2.000000000000003997 ) ;
#10972=ORIENTED_EDGE ( 'NONE', *, *, #7805, .T. ) ;
#10976=ORIENTED_EDGE ( 'NONE', *, *, #13080, .T. ) ;
#10978=AXIS2_PLACEMENT_3D ( 'NONE', #7039, #7952, #2900 ) ;
#10980=FACE_OUTER_BOUND ( 'NONE', #4131, .T. ) ;
#10988=ORIENTED_EDGE ( 'NONE', *, *, #5070, .T. ) ;
#10994=AXIS2_PLACEMENT_3D ( 'NONE', #11117, #4810, #9226 ) ;
#10995=CARTESIAN_POINT ( 'NONE',  ( -34.26147919318643886, 108.1862277804541321, 0.7448039452652762682 ) ) ;
#10998=LINE ( 'NONE', #7314, #370 ) ;
#11000=ORIENTED_EDGE ( 'NONE', *, *, #2830, .F. ) ;
#11003=VERTEX_POINT ( 'NONE', #10748 ) ;
#11008=ORIENTED_EDGE ( 'NONE', *, *, #3203, .T. ) ;
#11028=AXIS2_PLACEMENT_3D ( 'NONE', #3607, #7893, #12175 ) ;
#11035=CARTESIAN_POINT ( 'NONE',  ( 34.31346379765670918, 108.0181378390413016, -1.328939170454190855 ) ) ;
#11036=DIRECTION ( 'NONE',  ( -0.8000000000000010436, 0.5999999999999985345, 0.000000000000000000 ) ) ;
#11044=DIRECTION ( 'NONE',  ( 0.000000000000000000, -1.000000000000000000, 0.000000000000000000 ) ) ;
#11053=VERTEX_POINT ( 'NONE', #8648 ) ;
#11054=LINE ( 'NONE', #4388, #7704 ) ;
#11055=CARTESIAN_POINT ( 'NONE',  ( -39.06230589874905235, 109.5835921350012825, 7.500000000000000000 ) ) ;
#11056=EDGE_CURVE ( 'NONE', #5338, #6314, #795, .T. ) ;
#11060=CIRCLE ( 'NONE', #12415, 72.49999999999998579 ) ;
#11074=CARTESIAN_POINT ( 'NONE',  ( 25.00000000000000355, 120.0000000000000142, 2.499999999999999556 ) ) ;
#11083=AXIS2_PLACEMENT_3D ( 'NONE', #3887, #10134, #8166 ) ;
#11089=FACE_OUTER_BOUND ( 'NONE', #4469, .T. ) ;
#11101=ORIENTED_EDGE ( 'NONE', *, *, #3955, .F. ) ;
#11107=CARTESIAN_POINT ( 'NONE',  ( 35.20000000000002416, 106.4000000000000057, 2.500000000000000000 ) ) ;
#11115=AXIS2_PLACEMENT_3D ( 'NONE', #5024, #2921, #4884 ) ;
#11117=CARTESIAN_POINT ( 'NONE',  ( 0.000000000000000000, 71.01020514433645303, -7.500000000000000000 ) ) ;
#11118=DIRECTION ( 'NONE',  ( 0.000000000000000000, 0.000000000000000000, 1.000000000000000000 ) ) ;
#11121=CARTESIAN_POINT ( 'NONE',  ( 25.00000000000000355, 120.0000000000000142, 7.500000000000000000 ) ) ;
#11122=AXIS2_PLACEMENT_3D ( 'NONE', #3326, #3259, #9788 ) ;
#11131=LINE ( 'NONE', #8804, #6154 ) ;
#11133=EDGE_LOOP ( 'NONE', ( #6868, #4516, #10050, #12902, #6428, #3331 ) ) ;
#11158=EDGE_CURVE ( 'NONE', #10350, #214, #10646, .T. ) ;
#11159=DIRECTION ( 'NONE',  ( 0.000000000000000000, 0.000000000000000000, 1.000000000000000000 ) ) ;
#11168=DIRECTION ( 'NONE',  ( 0.000000000000000000, 0.000000000000000000, 1.000000000000000000 ) ) ;
#11175=ORIENTED_EDGE ( 'NONE', *, *, #4980, .T. ) ;
#11182=DIRECTION ( 'NONE',  ( 0.000000000000000000, 0.000000000000000000, 1.000000000000000000 ) ) ;
#11190=PLANE ( 'NONE',  #13705 ) ;
#11191=CARTESIAN_POINT ( 'NONE',  ( -40.73187278757662000, 100.6589795836331973, -1.037129925556720123 ) ) ;
#11192=CARTESIAN_POINT ( 'NONE',  ( 25.00000000000000355, 120.0000000000000142, -2.499999999999998668 ) ) ;
#11200=ORIENTED_EDGE ( 'NONE', *, *, #8076, .T. ) ;
#11201=DIRECTION ( 'NONE',  ( 1.000000000000000000, 0.000000000000000000, 0.000000000000000000 ) ) ;
#11204=CIRCLE ( 'NONE', #8723, 24.99999999999998934 ) ;
#11206=DIRECTION ( 'NONE',  ( -0.000000000000000000, 0.000000000000000000, 1.000000000000000000 ) ) ;
#11211=DIRECTION ( 'NONE',  ( 0.000000000000000000, 0.000000000000000000, 1.000000000000000000 ) ) ;
#11214=CIRCLE ( 'NONE', #1347, 5.000000000000004441 ) ;
#11224=VECTOR ( 'NONE', #9230, 1000.000000000000000 ) ;
#11227=CIRCLE ( 'NONE', #12115, 79.99999999999997158 ) ;
#11231=ORIENTED_EDGE ( 'NONE', *, *, #9635, .F. ) ;
#11234=VERTEX_POINT ( 'NONE', #9079 ) ;
#11235=DIRECTION ( 'NONE',  ( 1.000000000000000000, 0.000000000000000000, 0.000000000000000000 ) ) ;
#11236=( LENGTH_UNIT ( ) NAMED_UNIT ( * ) SI_UNIT ( .MILLI., .METRE. ) );
#11244=EDGE_CURVE ( 'NONE', #13844, #214, #3705, .T. ) ;
#11271=CARTESIAN_POINT ( 'NONE',  ( 25.00000000000000355, 120.0000000000000142, 7.500000000000000000 ) ) ;
#11283=VERTEX_POINT ( 'NONE', #7106 ) ;
#11310=AXIS2_PLACEMENT_3D ( 'NONE', #2335, #1289, #5493 ) ;
#11325=LINE ( 'NONE', #3823, #4642 ) ;
#11332=CIRCLE ( 'NONE', #9994, 22.49999999999998934 ) ;
#11334=EDGE_CURVE ( 'NONE', #6075, #1961, #3246, .T. ) ;
#11335=ORIENTED_EDGE ( 'NONE', *, *, #139, .F. ) ;
#11351=ORIENTED_EDGE ( 'NONE', *, *, #2590, .F. ) ;
#11361=VERTEX_POINT ( 'NONE', #4791 ) ;
#11366=CARTESIAN_POINT ( 'NONE',  ( -35.45454545454546036, 140.4866414850956744, -2.500000000000000000 ) ) ;
#11372=DIRECTION ( 'NONE',  ( 1.000000000000000000, 1.850371707708595154E-15, 0.000000000000000000 ) ) ;
#11373=ORIENTED_EDGE ( 'NONE', *, *, #892, .T. ) ;
#11379=AXIS2_PLACEMENT_3D ( 'NONE', #7496, #11840, #2367 ) ;
#11381=CARTESIAN_POINT ( 'NONE',  ( -25.00000000000000355, 120.0000000000000142, 2.499999999999999556 ) ) ;
#11407=ADVANCED_FACE ( 'NONE', ( #5621 ), #12904, .F. ) ;
#11414=CIRCLE ( 'NONE', #12770, 5.000000000000004441 ) ;
#11417=CIRCLE ( 'NONE', #224, 27.49999999999999289 ) ;
#11420=AXIS2_PLACEMENT_3D ( 'NONE', #2499, #1441, #4298 ) ;
#11422=CARTESIAN_POINT ( 'NONE',  ( 34.26155123102906686, 108.1859746833188041, 0.7471162051235300527 ) ) ;
#11437=ORIENTED_EDGE ( 'NONE', *, *, #9830, .F. ) ;
#11438=FACE_OUTER_BOUND ( 'NONE', #5824, .T. ) ;
#11444=AXIS2_PLACEMENT_3D ( 'NONE', #13125, #3480, #5384 ) ;
#11446=AXIS2_PLACEMENT_3D ( 'NONE', #9422, #13735, #648 ) ;
#11451=ORIENTED_EDGE ( 'NONE', *, *, #1370, .F. ) ;
#11468=EDGE_LOOP ( 'NONE', ( #3612, #734, #110, #7760 ) ) ;
#11474=CARTESIAN_POINT ( 'NONE',  ( 25.00000000000000355, 120.0000000000000142, 7.500000000000000000 ) ) ;
#11479=CARTESIAN_POINT ( 'NONE',  ( -39.99999999999999289, 120.0000000000000142, 0.5000000000000000000 ) ) ;
#11506=DIRECTION ( 'NONE',  ( -0.000000000000000000, -0.000000000000000000, -1.000000000000000000 ) ) ;
#11537=DIRECTION ( 'NONE',  ( 0.000000000000000000, 0.000000000000000000, 1.000000000000000000 ) ) ;
#11542=VERTEX_POINT ( 'NONE', #12504 ) ;
#11547=PLANE ( 'NONE',  #4044 ) ;
#11553=AXIS2_PLACEMENT_3D ( 'NONE', #3582, #2687, #12152 ) ;
#11566=DIRECTION ( 'NONE',  ( 1.000000000000000000, 0.000000000000000000, 0.000000000000000000 ) ) ;
#11571=CIRCLE ( 'NONE', #6641, 5.000000000000004441 ) ;
#11596=CARTESIAN_POINT ( 'NONE',  ( 35.45454545454547457, 140.4866414850956460, -2.500000000000000000 ) ) ;
#11604=ORIENTED_EDGE ( 'NONE', *, *, #7624, .F. ) ;
#11606=EDGE_CURVE ( 'NONE', #8180, #3641, #11994, .T. ) ;
#11616=B_SPLINE_CURVE_WITH_KNOTS ( 'NONE', 3,
 ( #12485, #3005, #11623, #7337, #9464, #9252, #13639, #13567, #13772, #772, #10371, #7144, #2945, #8465, #7277, #11422, #10502, #7210 ),
 .UNSPECIFIED., .F., .F.,
 ( 4, 2, 2, 2, 2, 2, 2, 2, 4 ),
 ( 2.478944061730947031E-07, 0.0003651306916264191360, 0.0007300134888466652469, 0.001094896286066911412, 0.001459779083287157360, 0.001824661880507403309, 0.002189544677727649474, 0.002554427474947895422, 0.002919310272168141370 ),
 .UNSPECIFIED. ) ;
#11618=ORIENTED_EDGE ( 'NONE', *, *, #13073, .F. ) ;
#11619=ORIENTED_EDGE ( 'NONE', *, *, #11244, .T. ) ;
#11623=CARTESIAN_POINT ( 'NONE',  ( 34.92076574184287097, 106.7798134293914103, 2.447438947438307810 ) ) ;
#11625=DIRECTION ( 'NONE',  ( -0.000000000000000000, -0.000000000000000000, -1.000000000000000000 ) ) ;
#11626=CARTESIAN_POINT ( 'NONE',  ( 25.00000000000000355, 120.0000000000000142, -7.500000000000000000 ) ) ;
#11642=CARTESIAN_POINT ( 'NONE',  ( 39.95750226049204912, 100.9609979968138731, -2.096206072712051949 ) ) ;
#11643=CARTESIAN_POINT ( 'NONE',  ( -35.22727272727274794, 140.0412797136805523, -2.499999999999999556 ) ) ;
#11651=ORIENTED_EDGE ( 'NONE', *, *, #10243, .T. ) ;
#11660=CIRCLE ( 'NONE', #9428, 4.999999999999998224 ) ;
#11664=DIRECTION ( 'NONE',  ( -0.6466635011015190448, 0.7627754036039218200, -0.000000000000000000 ) ) ;
#11665=EDGE_CURVE ( 'NONE', #4214, #7167, #4613, .T. ) ;
#11666=LINE ( 'NONE', #2057, #4606 ) ;
#11669=VECTOR ( 'NONE', #13088, 999.9999999999998863 ) ;
#11673=EDGE_CURVE ( 'NONE', #6752, #5579, #1744, .T. ) ;
#11674=ORIENTED_EDGE ( 'NONE', *, *, #289, .T. ) ;
#11677=EDGE_CURVE ( 'NONE', #4883, #2829, #10263, .T. ) ;
#11702=CARTESIAN_POINT ( 'NONE',  ( -45.50000000000000711, 101.0000000000000000, -7.500000000000000000 ) ) ;
#11705=FACE_OUTER_BOUND ( 'NONE', #2381, .T. ) ;
#11706=VERTEX_POINT ( 'NONE', #8000 ) ;
#11710=CARTESIAN_POINT ( 'NONE',  ( 38.89115197531749857, 101.6687180808697377, -2.500000000000000000 ) ) ;
#11712=AXIS2_PLACEMENT_3D ( 'NONE', #5459, #365, #8824 ) ;
#11719=AXIS2_PLACEMENT_3D ( 'NONE', #6273, #10940, #2188 ) ;
#11730=CARTESIAN_POINT ( 'NONE',  ( 35.04450421339217314, 112.5597086678580609, 2.499999999999999556 ) ) ;
#11732=ADVANCED_FACE ( 'NONE', ( #2522 ), #3477, .T. ) ;
#11739=AXIS2_PLACEMENT_3D ( 'NONE', #6434, #10697, #1109 ) ;
#11743=FACE_OUTER_BOUND ( 'NONE', #1268, .T. ) ;
#11749=CARTESIAN_POINT ( 'NONE',  ( 45.49999999999999289, 101.0000000000000142, 2.499999999999999556 ) ) ;
#11761=DIRECTION ( 'NONE',  ( -0.8000000000000008216, 0.5999999999999988676, 0.000000000000000000 ) ) ;
#11773=SPHERICAL_SURFACE ( 'NONE', #8969, 5.000000000000000000 ) ;
#11774=ORIENTED_EDGE ( 'NONE', *, *, #11673, .F. ) ;
#11784=ORIENTED_EDGE ( 'NONE', *, *, #7382, .T. ) ;
#11796=CARTESIAN_POINT ( 'NONE',  ( 32.72727272727274084, 135.1423002281141805, -2.500000000000000000 ) ) ;
#11800=DIRECTION ( 'NONE',  ( 1.000000000000000000, 0.000000000000000000, 0.000000000000000000 ) ) ;
#11809=EDGE_CURVE ( 'NONE', #3010, #769, #4378, .T. ) ;
#11811=DIRECTION ( 'NONE',  ( 0.000000000000000000, 0.000000000000000000, 1.000000000000000000 ) ) ;
#11814=CARTESIAN_POINT ( 'NONE',  ( 40.50666510048448288, 100.7305537260640307, 1.531269357928750185 ) ) ;
#11816=DIRECTION ( 'NONE',  ( 0.000000000000000000, 0.000000000000000000, 1.000000000000000000 ) ) ;
#11823=EDGE_CURVE ( 'NONE', #9570, #10854, #2887, .T. ) ;
#11825=ADVANCED_FACE ( 'NONE', ( #8063 ), #6107, .T. ) ;
#11828=DIRECTION ( 'NONE',  ( -0.000000000000000000, -0.000000000000000000, -1.000000000000000000 ) ) ;
#11840=DIRECTION ( 'NONE',  ( 0.000000000000000000, 0.000000000000000000, 1.000000000000000000 ) ) ;
#11842=CARTESIAN_POINT ( 'NONE',  ( -35.22727272727274794, 140.0412797136805523, 7.500000000000000000 ) ) ;
#11844=CARTESIAN_POINT ( 'NONE',  ( 40.24692185806991063, 100.8304034607652113, -1.836112450589440614 ) ) ;
#11851=ORIENTED_EDGE ( 'NONE', *, *, #1364, .T. ) ;
#11852=AXIS2_PLACEMENT_3D ( 'NONE', #10416, #1997, #7118 ) ;
#11859=AXIS2_PLACEMENT_3D ( 'NONE', #3751, #9151, #3676 ) ;
#11865=CIRCLE ( 'NONE', #2453, 24.99999999999998934 ) ;
#11867=CARTESIAN_POINT ( 'NONE',  ( -32.50000000000000000, 110.0000000000000142, -2.499999999999999556 ) ) ;
#11878=ORIENTED_EDGE ( 'NONE', *, *, #3773, .F. ) ;
#11879=CARTESIAN_POINT ( 'NONE',  ( 0.000000000000000000, 71.01020514433645303, -2.500000000000000000 ) ) ;
#11881=CARTESIAN_POINT ( 'NONE',  ( 34.40224804986664964, 107.7695571918731474, -1.740729949763267337 ) ) ;
#11883=DIRECTION ( 'NONE',  ( -0.4545454545454548634, 0.8907235428302464619, 0.000000000000000000 ) ) ;
#11884=DIRECTION ( 'NONE',  ( 1.000000000000000000, 0.000000000000000000, 0.000000000000000000 ) ) ;
#11885=CARTESIAN_POINT ( 'NONE',  ( 39.10039359579067764, 101.4951258812516812, 2.486679384192855835 ) ) ;
#11889=DIRECTION ( 'NONE',  ( -0.000000000000000000, -0.000000000000000000, -1.000000000000000000 ) ) ;
#11892=EDGE_LOOP ( 'NONE', ( #1888, #10704, #4092, #11200 ) ) ;
#11898=DIRECTION ( 'NONE',  ( -0.000000000000000000, -0.000000000000000000, -1.000000000000000000 ) ) ;
#11910=CARTESIAN_POINT ( 'NONE',  ( -34.33153323985096250, 107.9636705364999472, -1.438784920770796338 ) ) ;
#11914=AXIS2_PLACEMENT_3D ( 'NONE', #12893, #11811, #1294 ) ;
#11915=VERTEX_POINT ( 'NONE', #7078 ) ;
#11923=ORIENTED_EDGE ( 'NONE', *, *, #3172, .F. ) ;
#11924=DIRECTION ( 'NONE',  ( 1.000000000000000000, 0.000000000000000000, 0.000000000000000000 ) ) ;
#11946=DIRECTION ( 'NONE',  ( -0.000000000000000000, -0.000000000000000000, -1.000000000000000000 ) ) ;
#11948=CIRCLE ( 'NONE', #9500, 79.99999999999997158 ) ;
#11957=CIRCLE ( 'NONE', #7933, 16.99999999999998934 ) ;
#11966=CARTESIAN_POINT ( 'NONE',  ( 0.000000000000000000, 71.01020514433645303, -2.499999999999998668 ) ) ;
#11967=CARTESIAN_POINT ( 'NONE',  ( 25.00000000000000355, 120.0000000000000142, 2.499999999999999556 ) ) ;
#11968=CIRCLE ( 'NONE', #2121, 14.99999999999999112 ) ;
#11971=LINE ( 'NONE', #11702, #2722 ) ;
#11983=CARTESIAN_POINT ( 'NONE',  ( 25.00000000000000355, 120.0000000000000142, 2.500000000000000000 ) ) ;
#11988=ORIENTED_EDGE ( 'NONE', *, *, #1103, .F. ) ;
#11994=CIRCLE ( 'NONE', #5285, 4.999999999999997335 ) ;
#12003=DIRECTION ( 'NONE',  ( 1.000000000000000000, 0.000000000000000000, 0.000000000000000000 ) ) ;
#12004=EDGE_CURVE ( 'NONE', #13751, #3971, #8734, .T. ) ;
#12010=LINE ( 'NONE', #3244, #10297 ) ;
#12011=ORIENTED_EDGE ( 'NONE', *, *, #3508, .F. ) ;
#12018=CARTESIAN_POINT ( 'NONE',  ( 25.00000000000000355, 120.0000000000000142, -2.499999999999998668 ) ) ;
#12020=AXIS2_PLACEMENT_3D ( 'NONE', #12956, #3324, #11884 ) ;
#12021=CARTESIAN_POINT ( 'NONE',  ( -25.00000000000000355, 120.0000000000000142, 0.5000000000000000000 ) ) ;
#12024=CARTESIAN_POINT ( 'NONE',  ( -40.81228451836347659, 100.6358150620708471, -0.5000000000000000000 ) ) ;
#12026=EDGE_CURVE ( 'NONE', #7882, #13399, #10003, .T. ) ;
#12032=ORIENTED_EDGE ( 'NONE', *, *, #9712, .F. ) ;
#12058=ORIENTED_EDGE ( 'NONE', *, *, #11677, .T. ) ;
#12064=CARTESIAN_POINT ( 'NONE',  ( -25.00000000000000355, 120.0000000000000142, -2.499999999999998668 ) ) ;
#12071=DIRECTION ( 'NONE',  ( -0.000000000000000000, -0.000000000000000000, -1.000000000000000000 ) ) ;
#12082=EDGE_CURVE ( 'NONE', #5463, #6752, #5737, .T. ) ;
#12088=CARTESIAN_POINT ( 'NONE',  ( -37.50000000000000000, 120.0000000000000142, 7.500000000000000000 ) ) ;
#12089=ORIENTED_EDGE ( 'NONE', *, *, #11665, .F. ) ;
#12109=ADVANCED_FACE ( 'NONE', ( #8038 ), #1658, .T. ) ;
#12115=AXIS2_PLACEMENT_3D ( 'NONE', #2440, #7495, #1060 ) ;
#12118=CARTESIAN_POINT ( 'NONE',  ( 50.00000000000000000, 120.0000000000000142, 0.5000000000000000000 ) ) ;
#12127=DIRECTION ( 'NONE',  ( -0.6000000000000001998, -0.7999999999999998224, 0.000000000000000000 ) ) ;
#12129=ORIENTED_EDGE ( 'NONE', *, *, #1669, .T. ) ;
#12130=ORIENTED_EDGE ( 'NONE', *, *, #2795, .T. ) ;
#12131=FILL_AREA_STYLE ('',( #10168 ) ) ;
#12142=FACE_OUTER_BOUND ( 'NONE', #9374, .T. ) ;
#12152=DIRECTION ( 'NONE',  ( 0.6000000000000001998, 0.7999999999999999334, 0.000000000000000000 ) ) ;
#12157=VERTEX_POINT ( 'NONE', #5715 ) ;
#12163=AXIS2_PLACEMENT_3D ( 'NONE', #5166, #3910, #2857 ) ;
#12164=ORIENTED_EDGE ( 'NONE', *, *, #9467, .F. ) ;
#12166=EDGE_LOOP ( 'NONE', ( #5942, #7070, #9900, #10527, #10842, #2161, #5759, #13097 ) ) ;
#12175=DIRECTION ( 'NONE',  ( 1.000000000000000000, 0.000000000000000000, -0.000000000000000000 ) ) ;
#12186=DIRECTION ( 'NONE',  ( 1.000000000000000000, 0.000000000000000000, 0.000000000000000000 ) ) ;
#12189=ADVANCED_FACE ( 'NONE', ( #6009 ), #6843, .F. ) ;
#12197=CARTESIAN_POINT ( 'NONE',  ( 25.00000000000000355, 120.0000000000000142, -0.5000000000000000000 ) ) ;
#12198=ORIENTED_EDGE ( 'NONE', *, *, #2852, .F. ) ;
#12202=EDGE_LOOP ( 'NONE', ( #9862, #272, #9276, #9355 ) ) ;
#12209=CARTESIAN_POINT ( 'NONE',  ( -34.25812584745457201, 108.1980041606220908, 0.6234749816336021544 ) ) ;
#12221=DIRECTION ( 'NONE',  ( 0.000000000000000000, 0.000000000000000000, 1.000000000000000000 ) ) ;
#12225=CARTESIAN_POINT ( 'NONE',  ( -34.25812584745457201, 108.1980041606221192, -0.5000000000000000000 ) ) ;
#12232=ORIENTED_EDGE ( 'NONE', *, *, #1283, .F. ) ;
#12241=FACE_OUTER_BOUND ( 'NONE', #5132, .T. ) ;
#12243=TOROIDAL_SURFACE ( 'NONE', #13580, 22.49999999999999289, 5.000000000000000000 ) ;
#12247=CARTESIAN_POINT ( 'NONE',  ( 35.06230589874905945, 106.5835921350012825, 2.486789939184904874 ) ) ;
#12251=FACE_OUTER_BOUND ( 'NONE', #7082, .T. ) ;
#12252=ORIENTED_EDGE ( 'NONE', *, *, #480, .T. ) ;
#12267=FACE_OUTER_BOUND ( 'NONE', #4601, .T. ) ;
#12273=EDGE_CURVE ( 'NONE', #2573, #4214, #11948, .T. ) ;
#12277=CARTESIAN_POINT ( 'NONE',  ( 32.95454545454548878, 135.5876619995293026, -7.500000000000000000 ) ) ;
#12278=ORIENTED_EDGE ( 'NONE', *, *, #10243, .F. ) ;
#12288=( NAMED_UNIT ( * ) SI_UNIT ( $, .STERADIAN. ) SOLID_ANGLE_UNIT ( ) );
#12309=DIRECTION ( 'NONE',  ( 0.000000000000000000, 0.000000000000000000, -1.000000000000000000 ) ) ;
#12312=VECTOR ( 'NONE', #10601, 1000.000000000000000 ) ;
#12315=CARTESIAN_POINT ( 'NONE',  ( 34.06230589874904524, 109.5835921350012683, 2.499999999999999556 ) ) ;
#12322=EDGE_LOOP ( 'NONE', ( #10631, #2913, #11, #10852 ) ) ;
#12327=DIRECTION ( 'NONE',  ( 0.000000000000000000, 0.000000000000000000, 1.000000000000000000 ) ) ;
#12328=FACE_OUTER_BOUND ( 'NONE', #3757, .T. ) ;
#12336=EDGE_CURVE ( 'NONE', #11003, #4722, #1665, .T. ) ;
#12340=ORIENTED_EDGE ( 'NONE', *, *, #139, .T. ) ;
#12347=ORIENTED_EDGE ( 'NONE', *, *, #5247, .F. ) ;
#12353=EDGE_CURVE ( 'NONE', #9880, #4466, #4800, .T. ) ;
#12356=EDGE_CURVE ( 'NONE', #9516, #1913, #105, .T. ) ;
#12358=AXIS2_PLACEMENT_3D ( 'NONE', #5738, #2657, #3551 ) ;
#12359=EDGE_CURVE ( 'NONE', #9880, #10854, #3430, .T. ) ;
#12367=DIRECTION ( 'NONE',  ( -0.000000000000000000, -0.000000000000000000, -1.000000000000000000 ) ) ;
#12372=EDGE_CURVE ( 'NONE', #5632, #369, #8705, .T. ) ;
#12375=VERTEX_POINT ( 'NONE', #11730 ) ;
#12377=ORIENTED_EDGE ( 'NONE', *, *, #12082, .F. ) ;
#12378=EDGE_CURVE ( 'NONE', #13845, #11915, #6572, .T. ) ;
#12407=CARTESIAN_POINT ( 'NONE',  ( 42.16244658108817589, 105.4500712252157655, 2.499999999999999556 ) ) ;
#12408=DIRECTION ( 'NONE',  ( 0.4545454545454570283, 0.8907235428302452407, 0.000000000000000000 ) ) ;
#12413=( LENGTH_UNIT ( ) NAMED_UNIT ( * ) SI_UNIT ( .MILLI., .METRE. ) );
#12415=AXIS2_PLACEMENT_3D ( 'NONE', #10510, #5185, #8210 ) ;
#12421=ORIENTED_EDGE ( 'NONE', *, *, #9118, .F. ) ;
#12422=ADVANCED_FACE ( 'NONE', ( #2122 ), #8778, .T. ) ;
#12434=ORIENTED_EDGE ( 'NONE', *, *, #13403, .T. ) ;
#12437=CARTESIAN_POINT ( 'NONE',  ( 35.20000000000001705, 106.3999999999999915, -2.500000000000000000 ) ) ;
#12446=DIRECTION ( 'NONE',  ( 0.000000000000000000, 0.000000000000000000, -1.000000000000000000 ) ) ;
#12464=AXIS2_PLACEMENT_3D ( 'NONE', #1012, #2907, #1852 ) ;
#12465=EDGE_LOOP ( 'NONE', ( #4910, #4501, #9115, #12278, #10081, #13716, #9808, #5509, #11878, #13111, #4732, #7725 ) ) ;
#12467=DIRECTION ( 'NONE',  ( 1.000000000000000000, 0.000000000000000000, 0.000000000000000000 ) ) ;
#12485=CARTESIAN_POINT ( 'NONE',  ( 35.06230589874905945, 106.5835921350012825, 2.486789939184904874 ) ) ;
#12487=CARTESIAN_POINT ( 'NONE',  ( -34.91511737228312739, 106.7798435036222742, 2.458454180825600410 ) ) ;
#12497=DIRECTION ( 'NONE',  ( -1.000000000000000000, 0.000000000000000000, 0.000000000000000000 ) ) ;
#12500=( NAMED_UNIT ( * ) PLANE_ANGLE_UNIT ( ) SI_UNIT ( $, .RADIAN. ) );
#12504=CARTESIAN_POINT ( 'NONE',  ( 32.95454545454546036, 135.5876619995293026, 7.500000000000000000 ) ) ;
#12519=DIRECTION ( 'NONE',  ( -0.7999999999999999334, -0.6000000000000001998, 0.000000000000000000 ) ) ;
#12527=VECTOR ( 'NONE', #1413, 1000.000000000000000 ) ;
#12532=CARTESIAN_POINT ( 'NONE',  ( 42.16244658108818300, 105.4500712252157655, -2.499999999999998668 ) ) ;
#12553=ADVANCED_FACE ( 'NONE', ( #8929 ), #13232, .T. ) ;
#12560=CIRCLE ( 'NONE', #5392, 16.99999999999998934 ) ;
#12570=AXIS2_PLACEMENT_3D ( 'NONE', #8949, #13255, #6006 ) ;
#12574=ORIENTED_EDGE ( 'NONE', *, *, #8666, .F. ) ;
#12575=DIRECTION ( 'NONE',  ( 1.000000000000000000, 0.000000000000000000, 0.000000000000000000 ) ) ;
#12578=TOROIDAL_SURFACE ( 'NONE', #13725, 17.49999999999999289, 5.000000000000000000 ) ;
#12581=DIRECTION ( 'NONE',  ( -0.5952233065713573579, -0.8035603370713738647, 0.000000000000000000 ) ) ;
#12587=ORIENTED_EDGE ( 'NONE', *, *, #11158, .F. ) ;
#12588=EDGE_LOOP ( 'NONE', ( #13552, #3077, #10334, #12089 ) ) ;
#12596=DIRECTION ( 'NONE',  ( 0.000000000000000000, 0.000000000000000000, 1.000000000000000000 ) ) ;
#12606=EDGE_LOOP ( 'NONE', ( #10827, #7307, #12130, #11000 ) ) ;
#12607=DIRECTION ( 'NONE',  ( 0.000000000000000000, 0.000000000000000000, 1.000000000000000000 ) ) ;
#12623=EDGE_CURVE ( 'NONE', #5087, #1587, #5957, .T. ) ;
#12629=CARTESIAN_POINT ( 'NONE',  ( -35.04450421339218025, 112.5597086678580609, 7.500000000000000000 ) ) ;
#12647=AXIS2_PLACEMENT_3D ( 'NONE', #5623, #6474, #3240 ) ;
#12666=CARTESIAN_POINT ( 'NONE',  ( -25.00000000000000355, 120.0000000000000142, 0.5000000000000000000 ) ) ;
#12673=AXIS2_PLACEMENT_3D ( 'NONE', #3435, #5537, #10730 ) ;
#12678=FACE_OUTER_BOUND ( 'NONE', #1400, .T. ) ;
#12694=CARTESIAN_POINT ( 'NONE',  ( 25.00000000000000355, 120.0000000000000142, -0.5000000000000000000 ) ) ;
#12702=DIRECTION ( 'NONE',  ( -0.5999999999999982014, -0.8000000000000013767, -0.000000000000000000 ) ) ;
#12704=EDGE_CURVE ( 'NONE', #11706, #10135, #13820, .T. ) ;
#12707=AXIS2_PLACEMENT_3D ( 'NONE', #11749, #4439, #3391 ) ;
#12724=CARTESIAN_POINT ( 'NONE',  ( 25.00000000000000355, 120.0000000000000142, -2.499999999999998668 ) ) ;
#12726=DIRECTION ( 'NONE',  ( -0.000000000000000000, -0.000000000000000000, -1.000000000000000000 ) ) ;
#12750=ORIENTED_EDGE ( 'NONE', *, *, #2581, .F. ) ;
#12752=ORIENTED_EDGE ( 'NONE', *, *, #9256, .T. ) ;
#12756=AXIS2_PLACEMENT_3D ( 'NONE', #6396, #13666, #868 ) ;
#12770=AXIS2_PLACEMENT_3D ( 'NONE', #12532, #2064, #6276 ) ;
#12772=ORIENTED_EDGE ( 'NONE', *, *, #1503, .T. ) ;
#12775=DIRECTION ( 'NONE',  ( -0.7999999999999999334, -0.6000000000000001998, 0.000000000000000000 ) ) ;
#12779=CARTESIAN_POINT ( 'NONE',  ( 39.06230589874904524, 109.5835921350012683, 2.499999999999999556 ) ) ;
#12785=ORIENTED_EDGE ( 'NONE', *, *, #10493, .F. ) ;
#12790=ORIENTED_EDGE ( 'NONE', *, *, #3184, .T. ) ;
#12799=AXIS2_PLACEMENT_3D ( 'NONE', #5491, #115, #4367 ) ;
#12805=CARTESIAN_POINT ( 'NONE',  ( -42.16244658108818300, 105.4500712252157655, 2.499999999999999556 ) ) ;
#12808=EDGE_CURVE ( 'NONE', #1913, #10090, #2813, .T. ) ;
#12809=AXIS2_PLACEMENT_3D ( 'NONE', #13875, #10542, #8506 ) ;
#12810=VERTEX_POINT ( 'NONE', #7702 ) ;
#12814=ORIENTED_EDGE ( 'NONE', *, *, #11823, .T. ) ;
#12819=DIRECTION ( 'NONE',  ( 1.000000000000000000, 0.000000000000000000, 0.000000000000000000 ) ) ;
#12824=CIRCLE ( 'NONE', #44, 2.000000000000000000 ) ;
#12834=PRESENTATION_STYLE_ASSIGNMENT (( #972 ) ) ;
#12835=ORIENTED_EDGE ( 'NONE', *, *, #7624, .T. ) ;
#12836=CARTESIAN_POINT ( 'NONE',  ( 25.00000000000000355, 120.0000000000000142, 2.499999999999999556 ) ) ;
#12837=CARTESIAN_POINT ( 'NONE',  ( -35.20000000000000995, 106.3999999999999915, -0.5000000000000000000 ) ) ;
#12838=DIRECTION ( 'NONE',  ( 0.000000000000000000, 0.000000000000000000, 1.000000000000000000 ) ) ;
#12850=AXIS2_PLACEMENT_3D ( 'NONE', #7647, #10930, #11924 ) ;
#12853=DIRECTION ( 'NONE',  ( -0.000000000000000000, -0.000000000000000000, -1.000000000000000000 ) ) ;
#12857=DIRECTION ( 'NONE',  ( 1.000000000000000000, 0.000000000000000000, 0.000000000000000000 ) ) ;
#12863=AXIS2_PLACEMENT_3D ( 'NONE', #11121, #1508, #10068 ) ;
#12864=DIRECTION ( 'NONE',  ( -0.000000000000000000, -0.000000000000000000, -1.000000000000000000 ) ) ;
#12867=CYLINDRICAL_SURFACE ( 'NONE', #7972, 27.49999999999999289 ) ;
#12871=DIRECTION ( 'NONE',  ( 0.000000000000000000, 0.000000000000000000, -1.000000000000000000 ) ) ;
#12875=DIRECTION ( 'NONE',  ( -0.6000000000000001998, 0.7999999999999998224, -0.000000000000000000 ) ) ;
#12876=EDGE_CURVE ( 'NONE', #9459, #9003, #9752, .T. ) ;
#12886=AXIS2_PLACEMENT_3D ( 'NONE', #8452, #10814, #2337 ) ;
#12887=DIRECTION ( 'NONE',  ( 0.000000000000000000, 0.000000000000000000, 1.000000000000000000 ) ) ;
#12892=AXIS2_PLACEMENT_3D ( 'NONE', #2070, #8451, #1026 ) ;
#12893=CARTESIAN_POINT ( 'NONE',  ( -25.00000000000000355, 120.0000000000000142, 2.500000000000000000 ) ) ;
#12898=FACE_OUTER_BOUND ( 'NONE', #9504, .T. ) ;
#12902=ORIENTED_EDGE ( 'NONE', *, *, #406, .T. ) ;
#12904=TOROIDAL_SURFACE ( 'NONE', #8620, 77.99999999999997158, 2.000000000000000000 ) ;
#12905=DIRECTION ( 'NONE',  ( -0.000000000000000000, -0.000000000000000000, -1.000000000000000000 ) ) ;
#12910=CARTESIAN_POINT ( 'NONE',  ( -38.16244658108818300, 102.4500712252157797, -2.500000000000000444 ) ) ;
#12938=DIRECTION ( 'NONE',  ( 0.4545454545454548634, 0.8907235428302464619, 0.000000000000000000 ) ) ;
#12941=DIRECTION ( 'NONE',  ( 0.000000000000000000, 0.000000000000000000, 1.000000000000000000 ) ) ;
#12942=DIRECTION ( 'NONE',  ( 0.6000000000000001998, 0.7999999999999998224, -0.000000000000000000 ) ) ;
#12946=ORIENTED_EDGE ( 'NONE', *, *, #6719, .F. ) ;
#12950=DIRECTION ( 'NONE',  ( 0.000000000000000000, 0.000000000000000000, 1.000000000000000000 ) ) ;
#12956=CARTESIAN_POINT ( 'NONE',  ( -25.00000000000000355, 120.0000000000000142, -0.5000000000000000000 ) ) ;
#12966=( NAMED_UNIT ( * ) PLANE_ANGLE_UNIT ( ) SI_UNIT ( $, .RADIAN. ) );
#12969=ADVANCED_FACE ( 'NONE', ( #2447 ), #6405, .F. ) ;
#12971=EDGE_CURVE ( 'NONE', #2573, #8647, #10998, .T. ) ;
#12972=DIRECTION ( 'NONE',  ( -4.163336342344333082E-15, 1.000000000000000000, 1.734723475976805615E-16 ) ) ;
#12980=AXIS2_PLACEMENT_3D ( 'NONE', #9928, #13185, #13334 ) ;
#12988=CYLINDRICAL_SURFACE ( 'NONE', #10051, 24.99999999999998934 ) ;
#12998=ORIENTED_EDGE ( 'NONE', *, *, #6798, .F. ) ;
#13009=DIRECTION ( 'NONE',  ( 0.000000000000000000, 0.000000000000000000, 1.000000000000000000 ) ) ;
#13013=FACE_OUTER_BOUND ( 'NONE', #9749, .T. ) ;
#13016=AXIS2_PLACEMENT_3D ( 'NONE', #6997, #1670, #629 ) ;
#13025=CARTESIAN_POINT ( 'NONE',  ( 34.63132358390374321, 107.2645221665701456, -2.217002873864902135 ) ) ;
#13026=CIRCLE ( 'NONE', #12809, 27.49999999999998579 ) ;
#13034=CARTESIAN_POINT ( 'NONE',  ( 47.49999999999999289, 120.0000000000000142, -2.499999999999998668 ) ) ;
#13047=DIRECTION ( 'NONE',  ( 1.000000000000000000, 1.009293658750142794E-15, 0.000000000000000000 ) ) ;
#13055=EDGE_CURVE ( 'NONE', #10090, #6890, #11666, .T. ) ;
#13062=ADVANCED_FACE ( 'NONE', ( #10472 ), #4343, .F. ) ;
#13065=CARTESIAN_POINT ( 'NONE',  ( 39.10224891377572476, 101.4936815461678350, -2.486392430613897364 ) ) ;
#13073=EDGE_CURVE ( 'NONE', #9516, #6752, #2143, .T. ) ;
#13080=EDGE_CURVE ( 'NONE', #11053, #2573, #1704, .T. ) ;
#13082=CIRCLE ( 'NONE', #1641, 5.000000000000004441 ) ;
#13088=DIRECTION ( 'NONE',  ( 0.6000000000000001998, -0.7999999999999998224, -0.000000000000000000 ) ) ;
#13091=VECTOR ( 'NONE', #12942, 999.9999999999998863 ) ;
#13097=ORIENTED_EDGE ( 'NONE', *, *, #3023, .F. ) ;
#13105=DIRECTION ( 'NONE',  ( 0.000000000000000000, 0.000000000000000000, 1.000000000000000000 ) ) ;
#13111=ORIENTED_EDGE ( 'NONE', *, *, #5060, .F. ) ;
#13112=CARTESIAN_POINT ( 'NONE',  ( 35.06230589874905945, 106.5835921350012683, -2.499999999999999556 ) ) ;
#13117=VECTOR ( 'NONE', #4431, 1000.000000000000000 ) ;
#13125=CARTESIAN_POINT ( 'NONE',  ( -35.45454545454546036, 140.4866414850956460, 0.5000000000000000000 ) ) ;
#13139=EDGE_CURVE ( 'NONE', #369, #1961, #4037, .T. ) ;
#13150=DIRECTION ( 'NONE',  ( 0.000000000000000000, 0.000000000000000000, 1.000000000000000000 ) ) ;
#13158=AXIS2_PLACEMENT_3D ( 'NONE', #11055, #10012, #8966 ) ;
#13161=EDGE_CURVE ( 'NONE', #9616, #8450, #7733, .T. ) ;
#13175=AXIS2_PLACEMENT_3D ( 'NONE', #5871, #10144, #13407 ) ;
#13178=PRODUCT_DEFINITION_SHAPE ( 'NONE', 'NONE',  #4712 ) ;
#13179=DIRECTION ( 'NONE',  ( -0.6000000000000001998, 0.7999999999999998224, 0.000000000000000000 ) ) ;
#13185=DIRECTION ( 'NONE',  ( -0.8907235428302473501, -0.4545454545454531425, 0.000000000000000000 ) ) ;
#13186=ADVANCED_FACE ( 'NONE', ( #4957 ), #12243, .T. ) ;
#13187=EDGE_LOOP ( 'NONE', ( #8333, #9820, #13766, #3511, #3250, #6807, #12752, #13199, #13651, #5852 ) ) ;
#13191=ORIENTED_EDGE ( 'NONE', *, *, #5865, .T. ) ;
#13194=TOROIDAL_SURFACE ( 'NONE', #7995, 22.49999999999999289, 5.000000000000000000 ) ;
#13198=CARTESIAN_POINT ( 'NONE',  ( 42.16244658108817589, 105.4500712252157655, 7.500000000000000000 ) ) ;
#13199=ORIENTED_EDGE ( 'NONE', *, *, #9932, .T. ) ;
#13200=DIRECTION ( 'NONE',  ( 1.000000000000000000, 0.000000000000000000, 0.000000000000000000 ) ) ;
#13205=EDGE_LOOP ( 'NONE', ( #9707, #8144, #2402, #10988, #11674 ) ) ;
#13215=ORIENTED_EDGE ( 'NONE', *, *, #2363, .F. ) ;
#13221=EDGE_CURVE ( 'NONE', #8935, #11003, #11332, .T. ) ;
#13223=VERTEX_POINT ( 'NONE', #625 ) ;
#13232=PLANE ( 'NONE',  #11553 ) ;
#13233=ORIENTED_EDGE ( 'NONE', *, *, #13519, .T. ) ;
#13238=ORIENTED_EDGE ( 'NONE', *, *, #9562, .T. ) ;
#13240=EDGE_CURVE ( 'NONE', #6890, #12810, #6859, .T. ) ;
#13254=EDGE_CURVE ( 'NONE', #11542, #3469, #9763, .T. ) ;
#13255=DIRECTION ( 'NONE',  ( -0.000000000000000000, -0.000000000000000000, -1.000000000000000000 ) ) ;
#13259=PLANE ( 'NONE',  #11028 ) ;
#13267=ADVANCED_FACE ( 'NONE', ( #5292 ), #10556, .F. ) ;
#13276=FACE_OUTER_BOUND ( 'NONE', #3252, .T. ) ;
#13286=CARTESIAN_POINT ( 'NONE',  ( -34.25812584745457201, 108.1980041606221192, 0.5000000000000000000 ) ) ;
#13294=AXIS2_PLACEMENT_3D ( 'NONE', #8302, #12519, #6138 ) ;
#13295=CARTESIAN_POINT ( 'NONE',  ( -35.20000000000000995, 106.3999999999999915, 2.500000000000000000 ) ) ;
#13302=CARTESIAN_POINT ( 'NONE',  ( 25.00000000000000355, 120.0000000000000142, 0.5000000000000000000 ) ) ;
#13308=ORIENTED_EDGE ( 'NONE', *, *, #8360, .T. ) ;
#13311=CARTESIAN_POINT ( 'NONE',  ( -35.06230589874905235, 106.5835921350012825, -2.499999999999999556 ) ) ;
#13327=CARTESIAN_POINT ( 'NONE',  ( -39.95570474821490592, 100.9618745346225523, -2.097587229781390228 ) ) ;
#13329=CARTESIAN_POINT ( 'NONE',  ( 32.72727272727274084, 135.1423002281141805, -0.5000000000000000000 ) ) ;
#13333=CIRCLE ( 'NONE', #9041, 4.999999999999998224 ) ;
#13334=DIRECTION ( 'NONE',  ( 0.4545454545454531425, -0.8907235428302472391, 0.000000000000000000 ) ) ;
#13335=EDGE_CURVE ( 'NONE', #1662, #7167, #5280, .T. ) ;
#13341=ORIENTED_EDGE ( 'NONE', *, *, #13519, .F. ) ;
#13357=ADVANCED_FACE ( 'NONE', ( #11743 ), #7708, .T. ) ;
#13362=AXIS2_PLACEMENT_3D ( 'NONE', #4939, #10405, #10341 ) ;
#13367=ORIENTED_EDGE ( 'NONE', *, *, #5060, .T. ) ;
#13369=ORIENTED_EDGE ( 'NONE', *, *, #2737, .F. ) ;
#13373=ORIENTED_EDGE ( 'NONE', *, *, #8328, .F. ) ;
#13374=DIRECTION ( 'NONE',  ( 1.000000000000000000, 0.000000000000000000, 0.000000000000000000 ) ) ;
#13386=SPHERICAL_SURFACE ( 'NONE', #8683, 5.000000000000000000 ) ;
#13390=ORIENTED_EDGE ( 'NONE', *, *, #6341, .F. ) ;
#13394=AXIS2_PLACEMENT_3D ( 'NONE', #15, #3287, #7431 ) ;
#13395=DIRECTION ( 'NONE',  ( -0.8000000000000000444, 0.5999999999999999778, 0.000000000000000000 ) ) ;
#13396=MECHANICAL_DESIGN_GEOMETRIC_PRESENTATION_REPRESENTATION('',(#1702),#9761);
#13399=VERTEX_POINT ( 'NONE', #5354 ) ;
#13400=CARTESIAN_POINT ( 'NONE',  ( 47.49999999999999289, 120.0000000000000142, 2.499999999999999556 ) ) ;
#13403=EDGE_CURVE ( 'NONE', #2829, #11706, #11968, .T. ) ;
#13407=DIRECTION ( 'NONE',  ( -1.000000000000000000, 0.000000000000000000, 0.000000000000000000 ) ) ;
#13413=EDGE_LOOP ( 'NONE', ( #7364, #6115, #5112, #11604 ) ) ;
#13414=CIRCLE ( 'NONE', #3481, 16.99999999999998934 ) ;
#13427=ORIENTED_EDGE ( 'NONE', *, *, #8176, .T. ) ;
#13431=ORIENTED_EDGE ( 'NONE', *, *, #718, .T. ) ;
#13440=ORIENTED_EDGE ( 'NONE', *, *, #7382, .F. ) ;
#13448=SURFACE_SIDE_STYLE ('',( #9131 ) ) ;
#13459=CIRCLE ( 'NONE', #4901, 22.49999999999998934 ) ;
#13460=ORIENTED_EDGE ( 'NONE', *, *, #11809, .F. ) ;
#13466=DIRECTION ( 'NONE',  ( -0.5999999999999999778, -0.8000000000000000444, 0.000000000000000000 ) ) ;
#13467=DIRECTION ( 'NONE',  ( 0.4545454545454548634, 0.8907235428302464619, 0.000000000000000000 ) ) ;
#13468=ORIENTED_EDGE ( 'NONE', *, *, #6719, .T. ) ;
#13470=CARTESIAN_POINT ( 'NONE',  ( 42.49999999999999289, 120.0000000000000142, 2.499999999999999556 ) ) ;
#13474=LINE ( 'NONE', #7960, #7634 ) ;
#13478=DIRECTION ( 'NONE',  ( 1.000000000000000000, 0.000000000000000000, 0.000000000000000000 ) ) ;
#13491=CIRCLE ( 'NONE', #5837, 5.000000000000000888 ) ;
#13494=AXIS2_PLACEMENT_3D ( 'NONE', #6403, #4290, #8569 ) ;
#13495=CARTESIAN_POINT ( 'NONE',  ( 41.99999999999999289, 120.0000000000000142, -0.5000000000000000000 ) ) ;
#13503=AXIS2_PLACEMENT_3D ( 'NONE', #11381, #9285, #4868 ) ;
#13513=TOROIDAL_SURFACE ( 'NONE', #3150, 16.99999999999998934, 2.000000000000000000 ) ;
#13517=EDGE_CURVE ( 'NONE', #624, #1587, #1228, .T. ) ;
#13518=EDGE_CURVE ( 'NONE', #2025, #2515, #6759, .T. ) ;
#13519=EDGE_CURVE ( 'NONE', #7422, #8450, #10835, .T. ) ;
#13536=CARTESIAN_POINT ( 'NONE',  ( -40.81228451836347659, 100.6358150620708471, -0.5000000000000000000 ) ) ;
#13542=DIRECTION ( 'NONE',  ( 0.000000000000000000, 0.000000000000000000, 1.000000000000000000 ) ) ;
#13544=CARTESIAN_POINT ( 'NONE',  ( -38.16244658108818300, 102.4500712252157797, 2.499999999999999556 ) ) ;
#13547=AXIS2_PLACEMENT_3D ( 'NONE', #3275, #11828, #8809 ) ;
#13551=ADVANCED_FACE ( 'NONE', ( #4733 ), #5707, .T. ) ;
#13552=ORIENTED_EDGE ( 'NONE', *, *, #2071, .T. ) ;
#13561=ORIENTED_EDGE ( 'NONE', *, *, #9201, .F. ) ;
#13563=CARTESIAN_POINT ( 'NONE',  ( 42.16244658108818300, 105.4500712252157797, -7.500000000000000000 ) ) ;
#13567=CARTESIAN_POINT ( 'NONE',  ( 34.50158885938633802, 107.5319404580926630, 2.003700325319508035 ) ) ;
#13568=AXIS2_PLACEMENT_3D ( 'NONE', #7935, #587, #9127 ) ;
#13579=CYLINDRICAL_SURFACE ( 'NONE', #2228, 24.99999999999998934 ) ;
#13580=AXIS2_PLACEMENT_3D ( 'NONE', #8045, #12327, #6994 ) ;
#13593=ORIENTED_EDGE ( 'NONE', *, *, #1283, .T. ) ;
#13610=DIRECTION ( 'NONE',  ( 0.000000000000000000, 0.000000000000000000, -1.000000000000000000 ) ) ;
#13621=AXIS2_PLACEMENT_3D ( 'NONE', #12666, #5142, #9431 ) ;
#13626=EDGE_CURVE ( 'NONE', #3469, #9005, #1453, .T. ) ;
#13632=CARTESIAN_POINT ( 'NONE',  ( -29.00000000000000000, 123.0000000000000142, 7.500000000000000000 ) ) ;
#13639=CARTESIAN_POINT ( 'NONE',  ( 34.58461996471805122, 107.3565440455617477, 2.151643583074652977 ) ) ;
#13641=CARTESIAN_POINT ( 'NONE',  ( -34.58386302044580418, 107.3580618547655803, 2.150514425741564484 ) ) ;
#13644=ORIENTED_EDGE ( 'NONE', *, *, #2065, .F. ) ;
#13651=ORIENTED_EDGE ( 'NONE', *, *, #7288, .T. ) ;
#13659=ORIENTED_EDGE ( 'NONE', *, *, #7123, .T. ) ;
#13662=ADVANCED_FACE ( 'NONE', ( #2836 ), #8181, .F. ) ;
#13666=DIRECTION ( 'NONE',  ( -0.000000000000000000, -0.000000000000000000, -1.000000000000000000 ) ) ;
#13672=CARTESIAN_POINT ( 'NONE',  ( 48.00000000000000000, 120.0000000000000142, 0.5000000000000000000 ) ) ;
#13674=DIRECTION ( 'NONE',  ( 1.000000000000000000, 0.000000000000000000, 0.000000000000000000 ) ) ;
#13675=B_SPLINE_CURVE_WITH_KNOTS ( 'NONE', 3,
 ( #7061, #4604, #10085, #422, #3621, #8887, #4679, #3695, #5657, #7983, #499, #8048, #3840, #9168, #2794, #2508 ),
 .UNSPECIFIED., .F., .F.,
 ( 4, 2, 2, 2, 2, 2, 2, 4 ),
 ( 0.001123485749927461298, 0.001530777205506884606, 0.001938068661086307914, 0.002345360116665731222, 0.002752651572245154964, 0.003159943027824578272, 0.003567234483404001580, 0.004381817394562857737 ),
 .UNSPECIFIED. ) ;
#13684=ADVANCED_FACE ( 'NONE', ( #12241 ), #669, .T. ) ;
#13694=TOROIDAL_SURFACE ( 'NONE', #3791, 16.99999999999998934, 2.000000000000000000 ) ;
#13705=AXIS2_PLACEMENT_3D ( 'NONE', #747, #11118, #3603 ) ;
#13708=CARTESIAN_POINT ( 'NONE',  ( -35.45454545454546036, 140.4866414850956744, 2.500000000000000000 ) ) ;
#13716=ORIENTED_EDGE ( 'NONE', *, *, #1503, .F. ) ;
#13725=AXIS2_PLACEMENT_3D ( 'NONE', #11192, #7048, #4876 ) ;
#13727=CARTESIAN_POINT ( 'NONE',  ( 25.00000000000000355, 120.0000000000000142, -2.499999999999998668 ) ) ;
#13729=AXIS2_PLACEMENT_3D ( 'NONE', #4751, #3613, #2785 ) ;
#13735=DIRECTION ( 'NONE',  ( 1.077462011625539371E-16, -1.454589777793963520E-16, 1.000000000000000000 ) ) ;
#13736=AXIS2_PLACEMENT_3D ( 'NONE', #1920, #12596, #4085 ) ;
#13739=DIRECTION ( 'NONE',  ( -0.000000000000000000, -0.000000000000000000, -1.000000000000000000 ) ) ;
#13751=VERTEX_POINT ( 'NONE', #6135 ) ;
#13754=CARTESIAN_POINT ( 'NONE',  ( 25.00000000000000355, 120.0000000000000142, 2.499999999999999556 ) ) ;
#13760=EDGE_CURVE ( 'NONE', #2956, #11003, #8395, .T. ) ;
#13766=ORIENTED_EDGE ( 'NONE', *, *, #9271, .T. ) ;
#13772=CARTESIAN_POINT ( 'NONE',  ( 34.46489414126431683, 107.6161901685304372, 1.920132901535068326 ) ) ;
#13783=CARTESIAN_POINT ( 'NONE',  ( 0.000000000000000000, 71.01020514433645303, 2.499999999999999556 ) ) ;
#13794=EDGE_CURVE ( 'NONE', #8040, #6479, #6848, .T. ) ;
#13795=ORIENTED_EDGE ( 'NONE', *, *, #5666, .F. ) ;
#13816=ADVANCED_FACE ( 'NONE', ( #5339 ), #12867, .T. ) ;
#13818=ORIENTED_EDGE ( 'NONE', *, *, #13073, .T. ) ;
#13820=CIRCLE ( 'NONE', #9983, 14.99999999999999112 ) ;
#13834=( NAMED_UNIT ( * ) SI_UNIT ( $, .STERADIAN. ) SOLID_ANGLE_UNIT ( ) );
#13842=AXIS2_PLACEMENT_3D ( 'NONE', #1236, #5502, #187 ) ;
#13844=VERTEX_POINT ( 'NONE', #6330 ) ;
#13845=VERTEX_POINT ( 'NONE', #2112 ) ;
#13856=CARTESIAN_POINT ( 'NONE',  ( 39.42692690461820604, 101.2627928944373679, -2.396630853396261251 ) ) ;
#13859=CARTESIAN_POINT ( 'NONE',  ( 35.20000000000001705, 106.3999999999999915, -0.5000000000000000000 ) ) ;
#13873=CARTESIAN_POINT ( 'NONE',  ( -42.16244658108818300, 105.4500712252157655, 2.499999999999999556 ) ) ;
#13875=CARTESIAN_POINT ( 'NONE',  ( 25.00000000000000355, 120.0000000000000142, -2.499999999999998668 ) ) ;
#13876=DIRECTION ( 'NONE',  ( 1.000000000000000000, 3.469446951953615372E-15, 0.000000000000000000 ) ) ;
ENDSEC;
END-ISO-10303-21;
